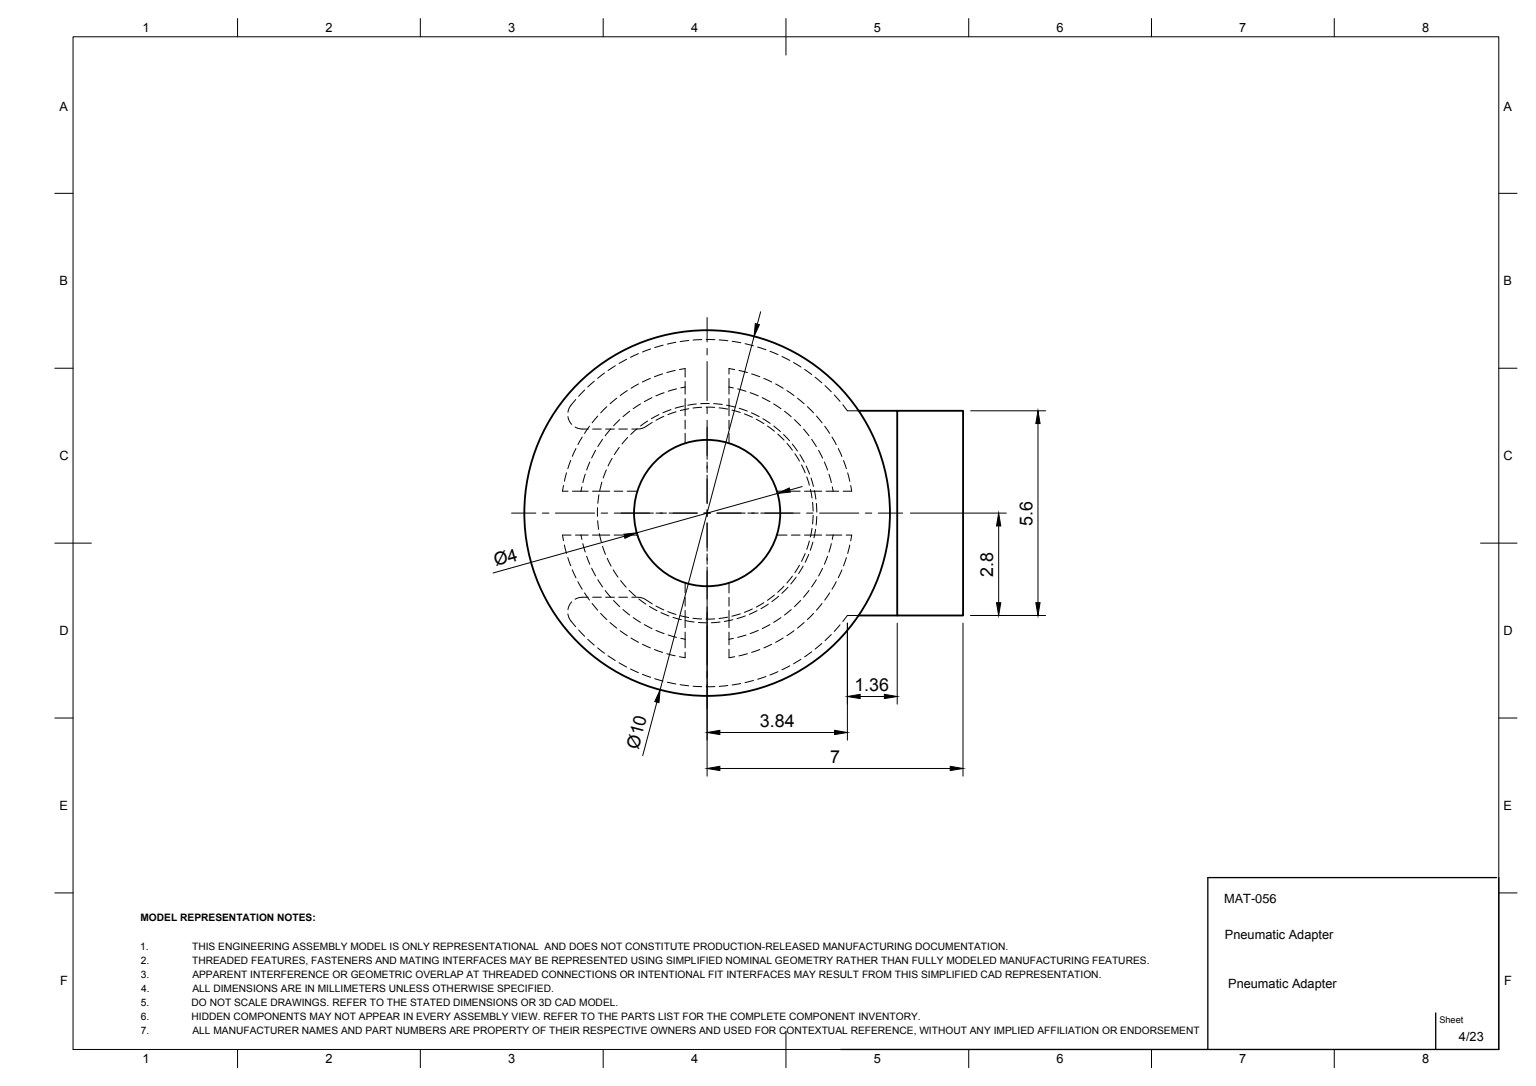
ISO-10303-21;
HEADER;
/* Generated by software containing ST-Developer
 * from STEP Tools, Inc. (www.steptools.com) 
 */

FILE_DESCRIPTION(
/* description */ (''),
/* implementation_level */ '2;1');

FILE_NAME(
/* name */ 'Pneumatic Adapter.step',
/* time_stamp */ '2026-10-28T16:47:13+01:00',
/* author */ (''),
/* organization */ (''),
/* preprocessor_version */ 'ST-DEVELOPER v20.2',
/* originating_system */ 'Autodesk Translation Framework v15.17.0.0',
/* authorisation */ '');

FILE_SCHEMA (('AUTOMOTIVE_DESIGN { 1 0 10303 214 3 1 1 }'));
ENDSEC;

DATA;
#10=MECHANICAL_DESIGN_GEOMETRIC_PRESENTATION_REPRESENTATION('',(#4567,#4568),#459242);
#4073=(
BOUNDED_CURVE()
B_SPLINE_CURVE(2,(#138438,#138439,#138440),.UNSPECIFIED.,.F.,.F.)
B_SPLINE_CURVE_WITH_KNOTS((3,3),(0.530296992815185,0.716353725522381),
 .UNSPECIFIED.)
CURVE()
GEOMETRIC_REPRESENTATION_ITEM()
RATIONAL_B_SPLINE_CURVE((1.02304101018598,1.02047479091633,1.01327152413875))
REPRESENTATION_ITEM('')
);
#4074=(
BOUNDED_CURVE()
B_SPLINE_CURVE(2,(#138443,#138444,#138445),.UNSPECIFIED.,.F.,.F.)
B_SPLINE_CURVE_WITH_KNOTS((3,3),(0.13830647491131,0.324363207617007),
 .UNSPECIFIED.)
CURVE()
GEOMETRIC_REPRESENTATION_ITEM()
RATIONAL_B_SPLINE_CURVE((1.01327152413597,1.02047479091208,1.02304101018125))
REPRESENTATION_ITEM('')
);
#4075=(
BOUNDED_CURVE()
B_SPLINE_CURVE(2,(#138448,#138449,#138450),.UNSPECIFIED.,.F.,.F.)
B_SPLINE_CURVE_WITH_KNOTS((3,3),(0.138306474911315,0.324363207616966),
 .UNSPECIFIED.)
CURVE()
GEOMETRIC_REPRESENTATION_ITEM()
RATIONAL_B_SPLINE_CURVE((1.01327152413589,1.02047479091195,1.02304101018111))
REPRESENTATION_ITEM('')
);
#4076=(
BOUNDED_CURVE()
B_SPLINE_CURVE(2,(#138452,#138453,#138454),.UNSPECIFIED.,.F.,.F.)
B_SPLINE_CURVE_WITH_KNOTS((3,3),(0.530296992818036,0.716353725523729),
 .UNSPECIFIED.)
CURVE()
GEOMETRIC_REPRESENTATION_ITEM()
RATIONAL_B_SPLINE_CURVE((1.02304101018115,1.02047479091198,1.01327152413591))
REPRESENTATION_ITEM('')
);
#4077=(
BOUNDED_CURVE()
B_SPLINE_CURVE(2,(#138458,#138459,#138460),.UNSPECIFIED.,.F.,.F.)
B_SPLINE_CURVE_WITH_KNOTS((3,3),(0.138306474911272,0.324363207616997),
 .UNSPECIFIED.)
CURVE()
GEOMETRIC_REPRESENTATION_ITEM()
RATIONAL_B_SPLINE_CURVE((1.01327152413612,1.02047479091231,1.02304101018152))
REPRESENTATION_ITEM('')
);
#4078=(
BOUNDED_CURVE()
B_SPLINE_CURVE(2,(#138462,#138463,#138464),.UNSPECIFIED.,.F.,.F.)
B_SPLINE_CURVE_WITH_KNOTS((3,3),(0.530296992818049,0.716353725523754),
 .UNSPECIFIED.)
CURVE()
GEOMETRIC_REPRESENTATION_ITEM()
RATIONAL_B_SPLINE_CURVE((1.0230410101813,1.02047479091212,1.013271524136))
REPRESENTATION_ITEM('')
);
#4079=(
BOUNDED_CURVE()
B_SPLINE_CURVE(2,(#138468,#138469,#138470),.UNSPECIFIED.,.F.,.F.)
B_SPLINE_CURVE_WITH_KNOTS((3,3),(1.87444128059995,1.89461071071013),
 .UNSPECIFIED.)
CURVE()
GEOMETRIC_REPRESENTATION_ITEM()
RATIONAL_B_SPLINE_CURVE((1.50304878048778,1.4222597775933,1.33967391292897))
REPRESENTATION_ITEM('')
);
#4080=(
BOUNDED_CURVE()
B_SPLINE_CURVE(2,(#138473,#138474,#138475),.UNSPECIFIED.,.F.,.F.)
B_SPLINE_CURVE_WITH_KNOTS((3,3),(0.0405896019330352,0.0607590320292299),
 .UNSPECIFIED.)
CURVE()
GEOMETRIC_REPRESENTATION_ITEM()
RATIONAL_B_SPLINE_CURVE((1.3396739130435,1.42225977764934,1.50304878048783))
REPRESENTATION_ITEM('')
);
#4081=(
BOUNDED_CURVE()
B_SPLINE_CURVE(2,(#138478,#138479,#138480),.UNSPECIFIED.,.F.,.F.)
B_SPLINE_CURVE_WITH_KNOTS((3,3),(0.0405896019330352,0.0607590320292299),
 .UNSPECIFIED.)
CURVE()
GEOMETRIC_REPRESENTATION_ITEM()
RATIONAL_B_SPLINE_CURVE((1.3396739130435,1.42225977764934,1.50304878048783))
REPRESENTATION_ITEM('')
);
#4082=(
BOUNDED_CURVE()
B_SPLINE_CURVE(2,(#138482,#138483,#138484),.UNSPECIFIED.,.F.,.F.)
B_SPLINE_CURVE_WITH_KNOTS((3,3),(1.87444128059996,1.89461071071012),
 .UNSPECIFIED.)
CURVE()
GEOMETRIC_REPRESENTATION_ITEM()
RATIONAL_B_SPLINE_CURVE((1.50304878048772,1.42225977759326,1.33967391292897))
REPRESENTATION_ITEM('')
);
#4083=(
BOUNDED_CURVE()
B_SPLINE_CURVE(2,(#138488,#138489,#138490),.UNSPECIFIED.,.F.,.F.)
B_SPLINE_CURVE_WITH_KNOTS((3,3),(0.0405896019330354,0.0607590320292301),
 .UNSPECIFIED.)
CURVE()
GEOMETRIC_REPRESENTATION_ITEM()
RATIONAL_B_SPLINE_CURVE((1.3396739130435,1.42225977764934,1.50304878048783))
REPRESENTATION_ITEM('')
);
#4084=(
BOUNDED_CURVE()
B_SPLINE_CURVE(2,(#138492,#138493,#138494),.UNSPECIFIED.,.F.,.F.)
B_SPLINE_CURVE_WITH_KNOTS((3,3),(1.87444128059996,1.89461071071014),
 .UNSPECIFIED.)
CURVE()
GEOMETRIC_REPRESENTATION_ITEM()
RATIONAL_B_SPLINE_CURVE((1.50304878048772,1.42225977759322,1.33967391292888))
REPRESENTATION_ITEM('')
);
#4085=(
BOUNDED_CURVE()
B_SPLINE_CURVE(2,(#138551,#138552,#138553),.UNSPECIFIED.,.F.,.F.)
B_SPLINE_CURVE_WITH_KNOTS((3,3),(0.530296992815185,0.716353725522381),
 .UNSPECIFIED.)
CURVE()
GEOMETRIC_REPRESENTATION_ITEM()
RATIONAL_B_SPLINE_CURVE((1.02304101018598,1.02047479091633,1.01327152413875))
REPRESENTATION_ITEM('')
);
#4086=(
BOUNDED_CURVE()
B_SPLINE_CURVE(2,(#138556,#138557,#138558),.UNSPECIFIED.,.F.,.F.)
B_SPLINE_CURVE_WITH_KNOTS((3,3),(0.13830647491131,0.324363207617007),
 .UNSPECIFIED.)
CURVE()
GEOMETRIC_REPRESENTATION_ITEM()
RATIONAL_B_SPLINE_CURVE((1.01327152413597,1.02047479091208,1.02304101018125))
REPRESENTATION_ITEM('')
);
#4087=(
BOUNDED_CURVE()
B_SPLINE_CURVE(2,(#138561,#138562,#138563),.UNSPECIFIED.,.F.,.F.)
B_SPLINE_CURVE_WITH_KNOTS((3,3),(1.87444128059995,1.89461071071013),
 .UNSPECIFIED.)
CURVE()
GEOMETRIC_REPRESENTATION_ITEM()
RATIONAL_B_SPLINE_CURVE((1.50304878048776,1.42225977759327,1.33967391292894))
REPRESENTATION_ITEM('')
);
#4088=(
BOUNDED_CURVE()
B_SPLINE_CURVE(2,(#138566,#138567,#138568),.UNSPECIFIED.,.F.,.F.)
B_SPLINE_CURVE_WITH_KNOTS((3,3),(0.0405896019330352,0.0607590320292299),
 .UNSPECIFIED.)
CURVE()
GEOMETRIC_REPRESENTATION_ITEM()
RATIONAL_B_SPLINE_CURVE((1.3396739130435,1.42225977764934,1.50304878048783))
REPRESENTATION_ITEM('')
);
#4406=SHAPE_REPRESENTATION_RELATIONSHIP('SRR','None',#459331,#4427);
#4427=ADVANCED_BREP_SHAPE_REPRESENTATION('',(#4448,#4449),#459220);
#4448=MANIFOLD_SOLID_BREP('Fitting body',#94624);
#4449=MANIFOLD_SOLID_BREP('Fixer',#94625);
#4567=STYLED_ITEM('',(#459519),#4448);
#4568=STYLED_ITEM('',(#459519),#4449);
#4664=CONICAL_SURFACE('',#95253,3.5,0.321750554396642);
#4665=CONICAL_SURFACE('',#95255,3.5,0.321750554396642);
#4666=CONICAL_SURFACE('',#95257,3.5,0.321750554396642);
#4667=CONICAL_SURFACE('',#95259,4.,0.558599315343569);
#4668=CONICAL_SURFACE('',#95261,4.,0.558599315343569);
#4669=CONICAL_SURFACE('',#95263,4.,0.558599315343569);
#4670=CONICAL_SURFACE('',#95281,3.5,0.321750554396642);
#4671=CONICAL_SURFACE('',#95283,4.,0.558599315343569);
#5124=FACE_BOUND('',#12374,.T.);
#5125=FACE_BOUND('',#12377,.T.);
#5321=PLANE('',#95244);
#5322=PLANE('',#95247);
#5323=PLANE('',#95250);
#5324=PLANE('',#95265);
#5325=PLANE('',#95267);
#5326=PLANE('',#95269);
#5327=PLANE('',#95279);
#5328=PLANE('',#95285);
#5329=PLANE('',#95294);
#5330=PLANE('',#95298);
#5331=PLANE('',#95299);
#5332=PLANE('',#95300);
#5333=PLANE('',#95301);
#5334=PLANE('',#95302);
#5335=PLANE('',#95303);
#5336=PLANE('',#95304);
#5337=PLANE('',#95305);
#5338=PLANE('',#95306);
#5339=PLANE('',#95307);
#5340=PLANE('',#95308);
#5341=PLANE('',#95309);
#5342=PLANE('',#95310);
#5343=PLANE('',#95314);
#5344=PLANE('',#95315);
#5345=PLANE('',#95334);
#5346=PLANE('',#95335);
#5347=PLANE('',#95336);
#5348=PLANE('',#95337);
#5349=PLANE('',#95338);
#5350=PLANE('',#95339);
#5351=PLANE('',#95340);
#6536=FACE_OUTER_BOUND('',#12355,.T.);
#6537=FACE_OUTER_BOUND('',#12356,.T.);
#6538=FACE_OUTER_BOUND('',#12357,.T.);
#6539=FACE_OUTER_BOUND('',#12358,.T.);
#6540=FACE_OUTER_BOUND('',#12359,.T.);
#6541=FACE_OUTER_BOUND('',#12360,.T.);
#6542=FACE_OUTER_BOUND('',#12361,.T.);
#6543=FACE_OUTER_BOUND('',#12362,.T.);
#6544=FACE_OUTER_BOUND('',#12363,.T.);
#6545=FACE_OUTER_BOUND('',#12364,.T.);
#6546=FACE_OUTER_BOUND('',#12365,.T.);
#6547=FACE_OUTER_BOUND('',#12366,.T.);
#6548=FACE_OUTER_BOUND('',#12367,.T.);
#6549=FACE_OUTER_BOUND('',#12368,.T.);
#6550=FACE_OUTER_BOUND('',#12369,.T.);
#6551=FACE_OUTER_BOUND('',#12370,.T.);
#6552=FACE_OUTER_BOUND('',#12371,.T.);
#6553=FACE_OUTER_BOUND('',#12372,.T.);
#6554=FACE_OUTER_BOUND('',#12373,.T.);
#6555=FACE_OUTER_BOUND('',#12375,.T.);
#6556=FACE_OUTER_BOUND('',#12376,.T.);
#6557=FACE_OUTER_BOUND('',#12378,.T.);
#6558=FACE_OUTER_BOUND('',#12379,.T.);
#6559=FACE_OUTER_BOUND('',#12380,.T.);
#6560=FACE_OUTER_BOUND('',#12381,.T.);
#6561=FACE_OUTER_BOUND('',#12382,.T.);
#6562=FACE_OUTER_BOUND('',#12383,.T.);
#6563=FACE_OUTER_BOUND('',#12384,.T.);
#6564=FACE_OUTER_BOUND('',#12385,.T.);
#6565=FACE_OUTER_BOUND('',#12386,.T.);
#6566=FACE_OUTER_BOUND('',#12387,.T.);
#6567=FACE_OUTER_BOUND('',#12388,.T.);
#6568=FACE_OUTER_BOUND('',#12389,.T.);
#6569=FACE_OUTER_BOUND('',#12390,.T.);
#6570=FACE_OUTER_BOUND('',#12391,.T.);
#6571=FACE_OUTER_BOUND('',#12392,.T.);
#6572=FACE_OUTER_BOUND('',#12393,.T.);
#6573=FACE_OUTER_BOUND('',#12394,.T.);
#6574=FACE_OUTER_BOUND('',#12395,.T.);
#6575=FACE_OUTER_BOUND('',#12396,.T.);
#6576=FACE_OUTER_BOUND('',#12397,.T.);
#6577=FACE_OUTER_BOUND('',#12398,.T.);
#6578=FACE_OUTER_BOUND('',#12399,.T.);
#6579=FACE_OUTER_BOUND('',#12400,.T.);
#6580=FACE_OUTER_BOUND('',#12401,.T.);
#6581=FACE_OUTER_BOUND('',#12402,.T.);
#6582=FACE_OUTER_BOUND('',#12403,.T.);
#6583=FACE_OUTER_BOUND('',#12404,.T.);
#6584=FACE_OUTER_BOUND('',#12405,.T.);
#12355=EDGE_LOOP('',(#59046,#59047,#59048,#59049));
#12356=EDGE_LOOP('',(#59050,#59051,#59052,#59053));
#12357=EDGE_LOOP('',(#59054,#59055,#59056,#59057));
#12358=EDGE_LOOP('',(#59058,#59059,#59060,#59061));
#12359=EDGE_LOOP('',(#59062,#59063,#59064,#59065));
#12360=EDGE_LOOP('',(#59066,#59067,#59068,#59069));
#12361=EDGE_LOOP('',(#59070,#59071,#59072,#59073));
#12362=EDGE_LOOP('',(#59074,#59075,#59076,#59077));
#12363=EDGE_LOOP('',(#59078,#59079,#59080,#59081));
#12364=EDGE_LOOP('',(#59082,#59083,#59084,#59085));
#12365=EDGE_LOOP('',(#59086,#59087,#59088,#59089));
#12366=EDGE_LOOP('',(#59090,#59091,#59092,#59093));
#12367=EDGE_LOOP('',(#59094,#59095,#59096,#59097,#59098,#59099,#59100,#59101,
#59102,#59103,#59104,#59105,#59106,#59107,#59108,#59109,#59110,#59111,#59112,
#59113));
#12368=EDGE_LOOP('',(#59114,#59115,#59116,#59117));
#12369=EDGE_LOOP('',(#59118,#59119,#59120,#59121));
#12370=EDGE_LOOP('',(#59122,#59123,#59124,#59125));
#12371=EDGE_LOOP('',(#59126,#59127,#59128,#59129));
#12372=EDGE_LOOP('',(#59130,#59131,#59132,#59133,#59134,#59135,#59136,#59137,
#59138,#59139,#59140,#59141,#59142,#59143,#59144,#59145,#59146,#59147,#59148,
#59149));
#12373=EDGE_LOOP('',(#59150));
#12374=EDGE_LOOP('',(#59151));
#12375=EDGE_LOOP('',(#59152,#59153,#59154,#59155));
#12376=EDGE_LOOP('',(#59156));
#12377=EDGE_LOOP('',(#59157));
#12378=EDGE_LOOP('',(#59158,#59159,#59160,#59161,#59162,#59163,#59164));
#12379=EDGE_LOOP('',(#59165,#59166,#59167,#59168,#59169,#59170,#59171));
#12380=EDGE_LOOP('',(#59172,#59173,#59174,#59175,#59176,#59177));
#12381=EDGE_LOOP('',(#59178,#59179,#59180,#59181,#59182,#59183,#59184));
#12382=EDGE_LOOP('',(#59185,#59186,#59187,#59188,#59189,#59190,#59191));
#12383=EDGE_LOOP('',(#59192,#59193,#59194,#59195));
#12384=EDGE_LOOP('',(#59196,#59197,#59198,#59199,#59200,#59201,#59202));
#12385=EDGE_LOOP('',(#59203,#59204,#59205,#59206,#59207,#59208,#59209));
#12386=EDGE_LOOP('',(#59210,#59211,#59212,#59213));
#12387=EDGE_LOOP('',(#59214,#59215,#59216,#59217,#59218,#59219,#59220));
#12388=EDGE_LOOP('',(#59221,#59222,#59223,#59224,#59225,#59226,#59227));
#12389=EDGE_LOOP('',(#59228,#59229,#59230,#59231));
#12390=EDGE_LOOP('',(#59232,#59233,#59234,#59235));
#12391=EDGE_LOOP('',(#59236,#59237,#59238,#59239));
#12392=EDGE_LOOP('',(#59240,#59241,#59242,#59243,#59244,#59245,#59246,#59247,
#59248,#59249,#59250,#59251));
#12393=EDGE_LOOP('',(#59252,#59253,#59254,#59255));
#12394=EDGE_LOOP('',(#59256,#59257,#59258,#59259));
#12395=EDGE_LOOP('',(#59260,#59261,#59262,#59263));
#12396=EDGE_LOOP('',(#59264,#59265,#59266,#59267));
#12397=EDGE_LOOP('',(#59268,#59269,#59270,#59271));
#12398=EDGE_LOOP('',(#59272,#59273,#59274,#59275));
#12399=EDGE_LOOP('',(#59276,#59277,#59278,#59279));
#12400=EDGE_LOOP('',(#59280,#59281,#59282,#59283));
#12401=EDGE_LOOP('',(#59284,#59285,#59286,#59287));
#12402=EDGE_LOOP('',(#59288,#59289,#59290,#59291,#59292,#59293));
#12403=EDGE_LOOP('',(#59294,#59295,#59296,#59297));
#12404=EDGE_LOOP('',(#59298,#59299,#59300,#59301,#59302,#59303));
#12405=EDGE_LOOP('',(#59304,#59305,#59306,#59307,#59308,#59309,#59310,#59311,
#59312,#59313,#59314,#59315));
#18307=CIRCLE('',#95245,3.5);
#18308=CIRCLE('',#95246,2.);
#18309=CIRCLE('',#95248,2.);
#18310=CIRCLE('',#95249,3.5);
#18311=CIRCLE('',#95251,2.);
#18312=CIRCLE('',#95252,3.5);
#18313=CIRCLE('',#95254,4.);
#18314=CIRCLE('',#95256,4.);
#18315=CIRCLE('',#95258,4.);
#18316=CIRCLE('',#95260,3.49999999999999);
#18317=CIRCLE('',#95262,3.49999999999999);
#18318=CIRCLE('',#95264,3.49999999999999);
#18319=CIRCLE('',#95266,3.);
#18320=CIRCLE('',#95268,3.);
#18321=CIRCLE('',#95270,3.);
#18322=CIRCLE('',#95272,2.);
#18323=CIRCLE('',#95273,2.);
#18324=CIRCLE('',#95274,2.);
#18325=CIRCLE('',#95275,2.);
#18326=CIRCLE('',#95276,2.);
#18327=CIRCLE('',#95277,2.);
#18328=CIRCLE('',#95278,2.);
#18329=CIRCLE('',#95280,3.5);
#18330=CIRCLE('',#95282,4.);
#18331=CIRCLE('',#95284,3.49999999999999);
#18332=CIRCLE('',#95286,3.);
#18333=CIRCLE('',#95288,3.);
#18334=CIRCLE('',#95289,3.);
#18335=CIRCLE('',#95290,3.);
#18336=CIRCLE('',#95291,3.);
#18337=CIRCLE('',#95292,3.);
#18338=CIRCLE('',#95293,3.);
#18339=CIRCLE('',#95295,5.);
#18340=CIRCLE('',#95297,5.);
#18341=CIRCLE('',#95312,0.4);
#18342=CIRCLE('',#95313,0.4);
#18343=CIRCLE('',#95316,2.9);
#18344=CIRCLE('',#95317,0.4);
#18345=CIRCLE('',#95318,0.4);
#18346=CIRCLE('',#95319,4.75);
#18347=CIRCLE('',#95320,4.75);
#18348=CIRCLE('',#95321,0.4);
#18349=CIRCLE('',#95323,0.4);
#18350=CIRCLE('',#95325,4.75);
#18351=CIRCLE('',#95327,0.4);
#18352=CIRCLE('',#95329,2.9);
#18353=CIRCLE('',#95331,0.4);
#18354=CIRCLE('',#95333,4.75);
#27269=LINE('',#138412,#31071);
#27270=LINE('',#138416,#31072);
#27271=LINE('',#138421,#31073);
#27272=LINE('',#138425,#31074);
#27273=LINE('',#138430,#31075);
#27274=LINE('',#138434,#31076);
#27275=LINE('',#138498,#31077);
#27276=LINE('',#138501,#31078);
#27277=LINE('',#138504,#31079);
#27278=LINE('',#138506,#31080);
#27279=LINE('',#138510,#31081);
#27280=LINE('',#138512,#31082);
#27281=LINE('',#138518,#31083);
#27282=LINE('',#138521,#31084);
#27283=LINE('',#138523,#31085);
#27284=LINE('',#138526,#31086);
#27285=LINE('',#138528,#31087);
#27286=LINE('',#138531,#31088);
#27287=LINE('',#138533,#31089);
#27288=LINE('',#138537,#31090);
#27289=LINE('',#138541,#31091);
#27290=LINE('',#138545,#31092);
#27291=LINE('',#138548,#31093);
#27292=LINE('',#138571,#31094);
#27293=LINE('',#138574,#31095);
#27294=LINE('',#138580,#31096);
#27295=LINE('',#138584,#31097);
#27296=LINE('',#138586,#31098);
#27297=LINE('',#138589,#31099);
#27298=LINE('',#138591,#31100);
#27299=LINE('',#138594,#31101);
#27300=LINE('',#138596,#31102);
#27301=LINE('',#138599,#31103);
#27302=LINE('',#138600,#31104);
#27303=LINE('',#138606,#31105);
#27304=LINE('',#138610,#31106);
#27305=LINE('',#138612,#31107);
#27306=LINE('',#138615,#31108);
#27307=LINE('',#138617,#31109);
#27308=LINE('',#138620,#31110);
#27309=LINE('',#138622,#31111);
#27310=LINE('',#138625,#31112);
#27311=LINE('',#138627,#31113);
#27312=LINE('',#138634,#31114);
#27313=LINE('',#138637,#31115);
#27314=LINE('',#138640,#31116);
#27315=LINE('',#138642,#31117);
#27316=LINE('',#138643,#31118);
#27317=LINE('',#138650,#31119);
#27318=LINE('',#138656,#31120);
#27319=LINE('',#138658,#31121);
#27320=LINE('',#138660,#31122);
#27321=LINE('',#138667,#31123);
#27322=LINE('',#138670,#31124);
#27323=LINE('',#138676,#31125);
#27324=LINE('',#138677,#31126);
#27325=LINE('',#138684,#31127);
#27326=LINE('',#138685,#31128);
#27327=LINE('',#138689,#31129);
#27328=LINE('',#138692,#31130);
#27329=LINE('',#138694,#31131);
#27330=LINE('',#138695,#31132);
#27331=LINE('',#138698,#31133);
#27332=LINE('',#138700,#31134);
#27333=LINE('',#138701,#31135);
#27334=LINE('',#138704,#31136);
#27335=LINE('',#138706,#31137);
#27336=LINE('',#138707,#31138);
#27337=LINE('',#138709,#31139);
#27338=LINE('',#138711,#31140);
#27339=LINE('',#138713,#31141);
#31071=VECTOR('',#106479,1000.);
#31072=VECTOR('',#106482,1000.);
#31073=VECTOR('',#106487,1000.);
#31074=VECTOR('',#106490,1000.);
#31075=VECTOR('',#106495,1000.);
#31076=VECTOR('',#106498,1000.);
#31077=VECTOR('',#106527,1000.);
#31078=VECTOR('',#106530,1000.);
#31079=VECTOR('',#106533,1000.);
#31080=VECTOR('',#106534,1000.);
#31081=VECTOR('',#106539,1000.);
#31082=VECTOR('',#106540,1000.);
#31083=VECTOR('',#106547,2.);
#31084=VECTOR('',#106550,1000.);
#31085=VECTOR('',#106551,1000.);
#31086=VECTOR('',#106554,1000.);
#31087=VECTOR('',#106555,1000.);
#31088=VECTOR('',#106558,1000.);
#31089=VECTOR('',#106559,1000.);
#31090=VECTOR('',#106562,1000.);
#31091=VECTOR('',#106565,1000.);
#31092=VECTOR('',#106570,1000.);
#31093=VECTOR('',#106573,1000.);
#31094=VECTOR('',#106584,1000.);
#31095=VECTOR('',#106587,1000.);
#31096=VECTOR('',#106592,3.);
#31097=VECTOR('',#106597,1000.);
#31098=VECTOR('',#106598,1000.);
#31099=VECTOR('',#106601,1000.);
#31100=VECTOR('',#106602,1000.);
#31101=VECTOR('',#106605,1000.);
#31102=VECTOR('',#106606,1000.);
#31103=VECTOR('',#106609,1000.);
#31104=VECTOR('',#106610,1000.);
#31105=VECTOR('',#106617,5.);
#31106=VECTOR('',#106624,1000.);
#31107=VECTOR('',#106627,1000.);
#31108=VECTOR('',#106632,1000.);
#31109=VECTOR('',#106635,1000.);
#31110=VECTOR('',#106640,1000.);
#31111=VECTOR('',#106643,1000.);
#31112=VECTOR('',#106648,1000.);
#31113=VECTOR('',#106651,1000.);
#31114=VECTOR('',#106658,10.);
#31115=VECTOR('',#106661,10.);
#31116=VECTOR('',#106664,10.);
#31117=VECTOR('',#106665,10.);
#31118=VECTOR('',#106666,10.);
#31119=VECTOR('',#106673,10.);
#31120=VECTOR('',#106678,10.);
#31121=VECTOR('',#106679,10.);
#31122=VECTOR('',#106680,10.);
#31123=VECTOR('',#106689,10.);
#31124=VECTOR('',#106692,10.);
#31125=VECTOR('',#106699,10.);
#31126=VECTOR('',#106700,10.);
#31127=VECTOR('',#106709,10.);
#31128=VECTOR('',#106710,10.);
#31129=VECTOR('',#106715,10.);
#31130=VECTOR('',#106718,10.);
#31131=VECTOR('',#106719,10.);
#31132=VECTOR('',#106720,10.);
#31133=VECTOR('',#106723,10.);
#31134=VECTOR('',#106724,10.);
#31135=VECTOR('',#106725,10.);
#31136=VECTOR('',#106728,10.);
#31137=VECTOR('',#106729,10.);
#31138=VECTOR('',#106730,10.);
#31139=VECTOR('',#106733,10.);
#31140=VECTOR('',#106736,10.);
#31141=VECTOR('',#106739,10.);
#34984=VERTEX_POINT('',#138410);
#34985=VERTEX_POINT('',#138411);
#34986=VERTEX_POINT('',#138413);
#34987=VERTEX_POINT('',#138415);
#34988=VERTEX_POINT('',#138419);
#34989=VERTEX_POINT('',#138420);
#34990=VERTEX_POINT('',#138422);
#34991=VERTEX_POINT('',#138424);
#34992=VERTEX_POINT('',#138428);
#34993=VERTEX_POINT('',#138429);
#34994=VERTEX_POINT('',#138431);
#34995=VERTEX_POINT('',#138433);
#34996=VERTEX_POINT('',#138437);
#34997=VERTEX_POINT('',#138441);
#34998=VERTEX_POINT('',#138447);
#34999=VERTEX_POINT('',#138451);
#35000=VERTEX_POINT('',#138457);
#35001=VERTEX_POINT('',#138461);
#35002=VERTEX_POINT('',#138467);
#35003=VERTEX_POINT('',#138471);
#35004=VERTEX_POINT('',#138477);
#35005=VERTEX_POINT('',#138481);
#35006=VERTEX_POINT('',#138487);
#35007=VERTEX_POINT('',#138491);
#35008=VERTEX_POINT('',#138497);
#35009=VERTEX_POINT('',#138499);
#35010=VERTEX_POINT('',#138503);
#35011=VERTEX_POINT('',#138505);
#35012=VERTEX_POINT('',#138509);
#35013=VERTEX_POINT('',#138511);
#35014=VERTEX_POINT('',#138515);
#35015=VERTEX_POINT('',#138517);
#35016=VERTEX_POINT('',#138519);
#35017=VERTEX_POINT('',#138522);
#35018=VERTEX_POINT('',#138524);
#35019=VERTEX_POINT('',#138527);
#35020=VERTEX_POINT('',#138529);
#35021=VERTEX_POINT('',#138532);
#35022=VERTEX_POINT('',#138534);
#35023=VERTEX_POINT('',#138536);
#35024=VERTEX_POINT('',#138538);
#35025=VERTEX_POINT('',#138540);
#35026=VERTEX_POINT('',#138544);
#35027=VERTEX_POINT('',#138546);
#35028=VERTEX_POINT('',#138550);
#35029=VERTEX_POINT('',#138554);
#35030=VERTEX_POINT('',#138560);
#35031=VERTEX_POINT('',#138564);
#35032=VERTEX_POINT('',#138570);
#35033=VERTEX_POINT('',#138572);
#35034=VERTEX_POINT('',#138576);
#35035=VERTEX_POINT('',#138577);
#35036=VERTEX_POINT('',#138579);
#35037=VERTEX_POINT('',#138582);
#35038=VERTEX_POINT('',#138585);
#35039=VERTEX_POINT('',#138587);
#35040=VERTEX_POINT('',#138590);
#35041=VERTEX_POINT('',#138592);
#35042=VERTEX_POINT('',#138595);
#35043=VERTEX_POINT('',#138597);
#35044=VERTEX_POINT('',#138602);
#35045=VERTEX_POINT('',#138605);
#35046=VERTEX_POINT('',#138630);
#35047=VERTEX_POINT('',#138631);
#35048=VERTEX_POINT('',#138633);
#35049=VERTEX_POINT('',#138635);
#35050=VERTEX_POINT('',#138639);
#35051=VERTEX_POINT('',#138641);
#35052=VERTEX_POINT('',#138645);
#35053=VERTEX_POINT('',#138647);
#35054=VERTEX_POINT('',#138649);
#35055=VERTEX_POINT('',#138651);
#35056=VERTEX_POINT('',#138653);
#35057=VERTEX_POINT('',#138655);
#35058=VERTEX_POINT('',#138657);
#35059=VERTEX_POINT('',#138659);
#35060=VERTEX_POINT('',#138661);
#35061=VERTEX_POINT('',#138665);
#35062=VERTEX_POINT('',#138669);
#35063=VERTEX_POINT('',#138673);
#35064=VERTEX_POINT('',#138674);
#35065=VERTEX_POINT('',#138681);
#35066=VERTEX_POINT('',#138682);
#35067=VERTEX_POINT('',#138687);
#35068=VERTEX_POINT('',#138691);
#35069=VERTEX_POINT('',#138693);
#35070=VERTEX_POINT('',#138697);
#35071=VERTEX_POINT('',#138699);
#35072=VERTEX_POINT('',#138703);
#35073=VERTEX_POINT('',#138705);
#44025=EDGE_CURVE('',#34984,#34985,#27269,.T.);
#44026=EDGE_CURVE('',#34984,#34986,#18307,.T.);
#44027=EDGE_CURVE('',#34987,#34986,#27270,.T.);
#44028=EDGE_CURVE('',#34985,#34987,#18308,.T.);
#44029=EDGE_CURVE('',#34988,#34989,#27271,.T.);
#44030=EDGE_CURVE('',#34990,#34988,#18309,.T.);
#44031=EDGE_CURVE('',#34991,#34990,#27272,.T.);
#44032=EDGE_CURVE('',#34991,#34989,#18310,.T.);
#44033=EDGE_CURVE('',#34992,#34993,#27273,.T.);
#44034=EDGE_CURVE('',#34994,#34992,#18311,.T.);
#44035=EDGE_CURVE('',#34995,#34994,#27274,.T.);
#44036=EDGE_CURVE('',#34995,#34993,#18312,.T.);
#44037=EDGE_CURVE('',#34996,#34984,#4073,.T.);
#44038=EDGE_CURVE('',#34996,#34997,#18313,.T.);
#44039=EDGE_CURVE('',#34986,#34997,#4074,.T.);
#44040=EDGE_CURVE('',#34989,#34998,#4075,.T.);
#44041=EDGE_CURVE('',#34999,#34991,#4076,.T.);
#44042=EDGE_CURVE('',#34999,#34998,#18314,.T.);
#44043=EDGE_CURVE('',#34993,#35000,#4077,.T.);
#44044=EDGE_CURVE('',#35001,#34995,#4078,.T.);
#44045=EDGE_CURVE('',#35001,#35000,#18315,.T.);
#44046=EDGE_CURVE('',#35002,#34996,#4079,.T.);
#44047=EDGE_CURVE('',#35002,#35003,#18316,.T.);
#44048=EDGE_CURVE('',#34997,#35003,#4080,.T.);
#44049=EDGE_CURVE('',#34998,#35004,#4081,.T.);
#44050=EDGE_CURVE('',#35005,#34999,#4082,.T.);
#44051=EDGE_CURVE('',#35005,#35004,#18317,.T.);
#44052=EDGE_CURVE('',#35000,#35006,#4083,.T.);
#44053=EDGE_CURVE('',#35007,#35001,#4084,.T.);
#44054=EDGE_CURVE('',#35007,#35006,#18318,.T.);
#44055=EDGE_CURVE('',#35008,#35002,#27275,.T.);
#44056=EDGE_CURVE('',#35008,#35009,#18319,.T.);
#44057=EDGE_CURVE('',#35003,#35009,#27276,.T.);
#44058=EDGE_CURVE('',#35004,#35010,#27277,.T.);
#44059=EDGE_CURVE('',#35011,#35005,#27278,.T.);
#44060=EDGE_CURVE('',#35011,#35010,#18320,.T.);
#44061=EDGE_CURVE('',#35006,#35012,#27279,.T.);
#44062=EDGE_CURVE('',#35013,#35007,#27280,.T.);
#44063=EDGE_CURVE('',#35013,#35012,#18321,.T.);
#44064=EDGE_CURVE('',#35014,#35014,#18322,.T.);
#44065=EDGE_CURVE('',#35014,#35015,#27281,.T.);
#44066=EDGE_CURVE('',#35015,#35016,#18323,.T.);
#44067=EDGE_CURVE('',#35016,#34994,#27282,.T.);
#44068=EDGE_CURVE('',#35017,#34992,#27283,.T.);
#44069=EDGE_CURVE('',#35017,#35018,#18324,.T.);
#44070=EDGE_CURVE('',#35018,#34990,#27284,.T.);
#44071=EDGE_CURVE('',#35019,#34988,#27285,.T.);
#44072=EDGE_CURVE('',#35019,#35020,#18325,.T.);
#44073=EDGE_CURVE('',#35020,#34985,#27286,.T.);
#44074=EDGE_CURVE('',#35021,#34987,#27287,.T.);
#44075=EDGE_CURVE('',#35021,#35022,#18326,.T.);
#44076=EDGE_CURVE('',#35022,#35023,#27288,.T.);
#44077=EDGE_CURVE('',#35023,#35024,#18327,.T.);
#44078=EDGE_CURVE('',#35025,#35024,#27289,.T.);
#44079=EDGE_CURVE('',#35025,#35015,#18328,.T.);
#44080=EDGE_CURVE('',#35026,#35023,#27290,.T.);
#44081=EDGE_CURVE('',#35026,#35027,#18329,.T.);
#44082=EDGE_CURVE('',#35024,#35027,#27291,.T.);
#44083=EDGE_CURVE('',#35028,#35026,#4085,.T.);
#44084=EDGE_CURVE('',#35028,#35029,#18330,.T.);
#44085=EDGE_CURVE('',#35027,#35029,#4086,.T.);
#44086=EDGE_CURVE('',#35030,#35028,#4087,.T.);
#44087=EDGE_CURVE('',#35030,#35031,#18331,.T.);
#44088=EDGE_CURVE('',#35029,#35031,#4088,.T.);
#44089=EDGE_CURVE('',#35032,#35030,#27292,.T.);
#44090=EDGE_CURVE('',#35032,#35033,#18332,.T.);
#44091=EDGE_CURVE('',#35031,#35033,#27293,.T.);
#44092=EDGE_CURVE('',#35034,#35035,#18333,.F.);
#44093=EDGE_CURVE('',#35035,#35036,#27294,.T.);
#44094=EDGE_CURVE('',#35036,#35036,#18334,.T.);
#44095=EDGE_CURVE('',#35035,#35037,#18335,.F.);
#44096=EDGE_CURVE('',#35033,#35037,#27295,.F.);
#44097=EDGE_CURVE('',#35038,#35032,#27296,.T.);
#44098=EDGE_CURVE('',#35038,#35039,#18336,.F.);
#44099=EDGE_CURVE('',#35009,#35039,#27297,.F.);
#44100=EDGE_CURVE('',#35040,#35008,#27298,.T.);
#44101=EDGE_CURVE('',#35040,#35041,#18337,.F.);
#44102=EDGE_CURVE('',#35010,#35041,#27299,.F.);
#44103=EDGE_CURVE('',#35042,#35011,#27300,.T.);
#44104=EDGE_CURVE('',#35042,#35043,#18338,.F.);
#44105=EDGE_CURVE('',#35012,#35043,#27301,.F.);
#44106=EDGE_CURVE('',#35034,#35013,#27302,.T.);
#44107=EDGE_CURVE('',#35044,#35044,#18339,.T.);
#44108=EDGE_CURVE('',#35044,#35045,#27303,.T.);
#44109=EDGE_CURVE('',#35045,#35045,#18340,.T.);
#44110=EDGE_CURVE('',#35037,#35025,#27304,.F.);
#44111=EDGE_CURVE('',#35016,#35034,#27305,.F.);
#44112=EDGE_CURVE('',#35039,#35021,#27306,.F.);
#44113=EDGE_CURVE('',#35022,#35038,#27307,.F.);
#44114=EDGE_CURVE('',#35018,#35042,#27308,.F.);
#44115=EDGE_CURVE('',#35043,#35017,#27309,.F.);
#44116=EDGE_CURVE('',#35020,#35040,#27310,.F.);
#44117=EDGE_CURVE('',#35041,#35019,#27311,.F.);
#44118=EDGE_CURVE('',#35046,#35047,#18341,.T.);
#44119=EDGE_CURVE('',#35047,#35048,#27312,.T.);
#44120=EDGE_CURVE('',#35048,#35049,#18342,.T.);
#44121=EDGE_CURVE('',#35049,#35046,#27313,.T.);
#44122=EDGE_CURVE('',#35049,#35050,#27314,.T.);
#44123=EDGE_CURVE('',#35051,#35050,#27315,.T.);
#44124=EDGE_CURVE('',#35046,#35051,#27316,.T.);
#44125=EDGE_CURVE('',#35048,#35052,#18343,.T.);
#44126=EDGE_CURVE('',#35053,#35052,#18344,.T.);
#44127=EDGE_CURVE('',#35053,#35054,#27317,.T.);
#44128=EDGE_CURVE('',#35055,#35054,#18345,.T.);
#44129=EDGE_CURVE('',#35056,#35055,#18346,.T.);
#44130=EDGE_CURVE('',#35057,#35056,#27318,.T.);
#44131=EDGE_CURVE('',#35057,#35058,#27319,.T.);
#44132=EDGE_CURVE('',#35058,#35059,#27320,.T.);
#44133=EDGE_CURVE('',#35060,#35059,#18347,.T.);
#44134=EDGE_CURVE('',#35050,#35060,#18348,.T.);
#44135=EDGE_CURVE('',#35061,#35051,#18349,.T.);
#44136=EDGE_CURVE('',#35060,#35061,#27321,.T.);
#44137=EDGE_CURVE('',#35059,#35062,#27322,.T.);
#44138=EDGE_CURVE('',#35061,#35062,#18350,.T.);
#44139=EDGE_CURVE('',#35063,#35064,#18351,.T.);
#44140=EDGE_CURVE('',#35064,#35053,#27323,.T.);
#44141=EDGE_CURVE('',#35052,#35063,#27324,.T.);
#44142=EDGE_CURVE('',#35063,#35047,#18352,.T.);
#44143=EDGE_CURVE('',#35065,#35066,#18353,.T.);
#44144=EDGE_CURVE('',#35066,#35055,#27325,.T.);
#44145=EDGE_CURVE('',#35054,#35065,#27326,.T.);
#44146=EDGE_CURVE('',#35067,#35066,#18354,.T.);
#44147=EDGE_CURVE('',#35056,#35067,#27327,.T.);
#44148=EDGE_CURVE('',#35057,#35068,#27328,.T.);
#44149=EDGE_CURVE('',#35069,#35068,#27329,.T.);
#44150=EDGE_CURVE('',#35058,#35069,#27330,.T.);
#44151=EDGE_CURVE('',#35068,#35070,#27331,.T.);
#44152=EDGE_CURVE('',#35070,#35071,#27332,.T.);
#44153=EDGE_CURVE('',#35071,#35069,#27333,.T.);
#44154=EDGE_CURVE('',#35072,#35070,#27334,.T.);
#44155=EDGE_CURVE('',#35073,#35072,#27335,.T.);
#44156=EDGE_CURVE('',#35071,#35073,#27336,.T.);
#44157=EDGE_CURVE('',#35062,#35073,#27337,.T.);
#44158=EDGE_CURVE('',#35065,#35064,#27338,.T.);
#44159=EDGE_CURVE('',#35072,#35067,#27339,.T.);
#59046=ORIENTED_EDGE('',*,*,#44025,.F.);
#59047=ORIENTED_EDGE('',*,*,#44026,.T.);
#59048=ORIENTED_EDGE('',*,*,#44027,.F.);
#59049=ORIENTED_EDGE('',*,*,#44028,.F.);
#59050=ORIENTED_EDGE('',*,*,#44029,.F.);
#59051=ORIENTED_EDGE('',*,*,#44030,.F.);
#59052=ORIENTED_EDGE('',*,*,#44031,.F.);
#59053=ORIENTED_EDGE('',*,*,#44032,.T.);
#59054=ORIENTED_EDGE('',*,*,#44033,.F.);
#59055=ORIENTED_EDGE('',*,*,#44034,.F.);
#59056=ORIENTED_EDGE('',*,*,#44035,.F.);
#59057=ORIENTED_EDGE('',*,*,#44036,.T.);
#59058=ORIENTED_EDGE('',*,*,#44037,.F.);
#59059=ORIENTED_EDGE('',*,*,#44038,.T.);
#59060=ORIENTED_EDGE('',*,*,#44039,.F.);
#59061=ORIENTED_EDGE('',*,*,#44026,.F.);
#59062=ORIENTED_EDGE('',*,*,#44040,.F.);
#59063=ORIENTED_EDGE('',*,*,#44032,.F.);
#59064=ORIENTED_EDGE('',*,*,#44041,.F.);
#59065=ORIENTED_EDGE('',*,*,#44042,.T.);
#59066=ORIENTED_EDGE('',*,*,#44043,.F.);
#59067=ORIENTED_EDGE('',*,*,#44036,.F.);
#59068=ORIENTED_EDGE('',*,*,#44044,.F.);
#59069=ORIENTED_EDGE('',*,*,#44045,.T.);
#59070=ORIENTED_EDGE('',*,*,#44046,.F.);
#59071=ORIENTED_EDGE('',*,*,#44047,.T.);
#59072=ORIENTED_EDGE('',*,*,#44048,.F.);
#59073=ORIENTED_EDGE('',*,*,#44038,.F.);
#59074=ORIENTED_EDGE('',*,*,#44049,.F.);
#59075=ORIENTED_EDGE('',*,*,#44042,.F.);
#59076=ORIENTED_EDGE('',*,*,#44050,.F.);
#59077=ORIENTED_EDGE('',*,*,#44051,.T.);
#59078=ORIENTED_EDGE('',*,*,#44052,.F.);
#59079=ORIENTED_EDGE('',*,*,#44045,.F.);
#59080=ORIENTED_EDGE('',*,*,#44053,.F.);
#59081=ORIENTED_EDGE('',*,*,#44054,.T.);
#59082=ORIENTED_EDGE('',*,*,#44055,.F.);
#59083=ORIENTED_EDGE('',*,*,#44056,.T.);
#59084=ORIENTED_EDGE('',*,*,#44057,.F.);
#59085=ORIENTED_EDGE('',*,*,#44047,.F.);
#59086=ORIENTED_EDGE('',*,*,#44058,.F.);
#59087=ORIENTED_EDGE('',*,*,#44051,.F.);
#59088=ORIENTED_EDGE('',*,*,#44059,.F.);
#59089=ORIENTED_EDGE('',*,*,#44060,.T.);
#59090=ORIENTED_EDGE('',*,*,#44061,.F.);
#59091=ORIENTED_EDGE('',*,*,#44054,.F.);
#59092=ORIENTED_EDGE('',*,*,#44062,.F.);
#59093=ORIENTED_EDGE('',*,*,#44063,.T.);
#59094=ORIENTED_EDGE('',*,*,#44064,.F.);
#59095=ORIENTED_EDGE('',*,*,#44065,.T.);
#59096=ORIENTED_EDGE('',*,*,#44066,.T.);
#59097=ORIENTED_EDGE('',*,*,#44067,.T.);
#59098=ORIENTED_EDGE('',*,*,#44034,.T.);
#59099=ORIENTED_EDGE('',*,*,#44068,.F.);
#59100=ORIENTED_EDGE('',*,*,#44069,.T.);
#59101=ORIENTED_EDGE('',*,*,#44070,.T.);
#59102=ORIENTED_EDGE('',*,*,#44030,.T.);
#59103=ORIENTED_EDGE('',*,*,#44071,.F.);
#59104=ORIENTED_EDGE('',*,*,#44072,.T.);
#59105=ORIENTED_EDGE('',*,*,#44073,.T.);
#59106=ORIENTED_EDGE('',*,*,#44028,.T.);
#59107=ORIENTED_EDGE('',*,*,#44074,.F.);
#59108=ORIENTED_EDGE('',*,*,#44075,.T.);
#59109=ORIENTED_EDGE('',*,*,#44076,.T.);
#59110=ORIENTED_EDGE('',*,*,#44077,.T.);
#59111=ORIENTED_EDGE('',*,*,#44078,.F.);
#59112=ORIENTED_EDGE('',*,*,#44079,.T.);
#59113=ORIENTED_EDGE('',*,*,#44065,.F.);
#59114=ORIENTED_EDGE('',*,*,#44080,.F.);
#59115=ORIENTED_EDGE('',*,*,#44081,.T.);
#59116=ORIENTED_EDGE('',*,*,#44082,.F.);
#59117=ORIENTED_EDGE('',*,*,#44077,.F.);
#59118=ORIENTED_EDGE('',*,*,#44083,.F.);
#59119=ORIENTED_EDGE('',*,*,#44084,.T.);
#59120=ORIENTED_EDGE('',*,*,#44085,.F.);
#59121=ORIENTED_EDGE('',*,*,#44081,.F.);
#59122=ORIENTED_EDGE('',*,*,#44086,.F.);
#59123=ORIENTED_EDGE('',*,*,#44087,.T.);
#59124=ORIENTED_EDGE('',*,*,#44088,.F.);
#59125=ORIENTED_EDGE('',*,*,#44084,.F.);
#59126=ORIENTED_EDGE('',*,*,#44089,.F.);
#59127=ORIENTED_EDGE('',*,*,#44090,.T.);
#59128=ORIENTED_EDGE('',*,*,#44091,.F.);
#59129=ORIENTED_EDGE('',*,*,#44087,.F.);
#59130=ORIENTED_EDGE('',*,*,#44092,.T.);
#59131=ORIENTED_EDGE('',*,*,#44093,.T.);
#59132=ORIENTED_EDGE('',*,*,#44094,.T.);
#59133=ORIENTED_EDGE('',*,*,#44093,.F.);
#59134=ORIENTED_EDGE('',*,*,#44095,.T.);
#59135=ORIENTED_EDGE('',*,*,#44096,.F.);
#59136=ORIENTED_EDGE('',*,*,#44090,.F.);
#59137=ORIENTED_EDGE('',*,*,#44097,.F.);
#59138=ORIENTED_EDGE('',*,*,#44098,.T.);
#59139=ORIENTED_EDGE('',*,*,#44099,.F.);
#59140=ORIENTED_EDGE('',*,*,#44056,.F.);
#59141=ORIENTED_EDGE('',*,*,#44100,.F.);
#59142=ORIENTED_EDGE('',*,*,#44101,.T.);
#59143=ORIENTED_EDGE('',*,*,#44102,.F.);
#59144=ORIENTED_EDGE('',*,*,#44060,.F.);
#59145=ORIENTED_EDGE('',*,*,#44103,.F.);
#59146=ORIENTED_EDGE('',*,*,#44104,.T.);
#59147=ORIENTED_EDGE('',*,*,#44105,.F.);
#59148=ORIENTED_EDGE('',*,*,#44063,.F.);
#59149=ORIENTED_EDGE('',*,*,#44106,.F.);
#59150=ORIENTED_EDGE('',*,*,#44107,.T.);
#59151=ORIENTED_EDGE('',*,*,#44094,.F.);
#59152=ORIENTED_EDGE('',*,*,#44107,.F.);
#59153=ORIENTED_EDGE('',*,*,#44108,.T.);
#59154=ORIENTED_EDGE('',*,*,#44109,.T.);
#59155=ORIENTED_EDGE('',*,*,#44108,.F.);
#59156=ORIENTED_EDGE('',*,*,#44109,.F.);
#59157=ORIENTED_EDGE('',*,*,#44064,.T.);
#59158=ORIENTED_EDGE('',*,*,#44085,.T.);
#59159=ORIENTED_EDGE('',*,*,#44088,.T.);
#59160=ORIENTED_EDGE('',*,*,#44091,.T.);
#59161=ORIENTED_EDGE('',*,*,#44096,.T.);
#59162=ORIENTED_EDGE('',*,*,#44110,.T.);
#59163=ORIENTED_EDGE('',*,*,#44078,.T.);
#59164=ORIENTED_EDGE('',*,*,#44082,.T.);
#59165=ORIENTED_EDGE('',*,*,#44044,.T.);
#59166=ORIENTED_EDGE('',*,*,#44035,.T.);
#59167=ORIENTED_EDGE('',*,*,#44067,.F.);
#59168=ORIENTED_EDGE('',*,*,#44111,.T.);
#59169=ORIENTED_EDGE('',*,*,#44106,.T.);
#59170=ORIENTED_EDGE('',*,*,#44062,.T.);
#59171=ORIENTED_EDGE('',*,*,#44053,.T.);
#59172=ORIENTED_EDGE('',*,*,#44110,.F.);
#59173=ORIENTED_EDGE('',*,*,#44095,.F.);
#59174=ORIENTED_EDGE('',*,*,#44092,.F.);
#59175=ORIENTED_EDGE('',*,*,#44111,.F.);
#59176=ORIENTED_EDGE('',*,*,#44066,.F.);
#59177=ORIENTED_EDGE('',*,*,#44079,.F.);
#59178=ORIENTED_EDGE('',*,*,#44039,.T.);
#59179=ORIENTED_EDGE('',*,*,#44048,.T.);
#59180=ORIENTED_EDGE('',*,*,#44057,.T.);
#59181=ORIENTED_EDGE('',*,*,#44099,.T.);
#59182=ORIENTED_EDGE('',*,*,#44112,.T.);
#59183=ORIENTED_EDGE('',*,*,#44074,.T.);
#59184=ORIENTED_EDGE('',*,*,#44027,.T.);
#59185=ORIENTED_EDGE('',*,*,#44083,.T.);
#59186=ORIENTED_EDGE('',*,*,#44080,.T.);
#59187=ORIENTED_EDGE('',*,*,#44076,.F.);
#59188=ORIENTED_EDGE('',*,*,#44113,.T.);
#59189=ORIENTED_EDGE('',*,*,#44097,.T.);
#59190=ORIENTED_EDGE('',*,*,#44089,.T.);
#59191=ORIENTED_EDGE('',*,*,#44086,.T.);
#59192=ORIENTED_EDGE('',*,*,#44112,.F.);
#59193=ORIENTED_EDGE('',*,*,#44098,.F.);
#59194=ORIENTED_EDGE('',*,*,#44113,.F.);
#59195=ORIENTED_EDGE('',*,*,#44075,.F.);
#59196=ORIENTED_EDGE('',*,*,#44041,.T.);
#59197=ORIENTED_EDGE('',*,*,#44031,.T.);
#59198=ORIENTED_EDGE('',*,*,#44070,.F.);
#59199=ORIENTED_EDGE('',*,*,#44114,.T.);
#59200=ORIENTED_EDGE('',*,*,#44103,.T.);
#59201=ORIENTED_EDGE('',*,*,#44059,.T.);
#59202=ORIENTED_EDGE('',*,*,#44050,.T.);
#59203=ORIENTED_EDGE('',*,*,#44043,.T.);
#59204=ORIENTED_EDGE('',*,*,#44052,.T.);
#59205=ORIENTED_EDGE('',*,*,#44061,.T.);
#59206=ORIENTED_EDGE('',*,*,#44105,.T.);
#59207=ORIENTED_EDGE('',*,*,#44115,.T.);
#59208=ORIENTED_EDGE('',*,*,#44068,.T.);
#59209=ORIENTED_EDGE('',*,*,#44033,.T.);
#59210=ORIENTED_EDGE('',*,*,#44115,.F.);
#59211=ORIENTED_EDGE('',*,*,#44104,.F.);
#59212=ORIENTED_EDGE('',*,*,#44114,.F.);
#59213=ORIENTED_EDGE('',*,*,#44069,.F.);
#59214=ORIENTED_EDGE('',*,*,#44037,.T.);
#59215=ORIENTED_EDGE('',*,*,#44025,.T.);
#59216=ORIENTED_EDGE('',*,*,#44073,.F.);
#59217=ORIENTED_EDGE('',*,*,#44116,.T.);
#59218=ORIENTED_EDGE('',*,*,#44100,.T.);
#59219=ORIENTED_EDGE('',*,*,#44055,.T.);
#59220=ORIENTED_EDGE('',*,*,#44046,.T.);
#59221=ORIENTED_EDGE('',*,*,#44040,.T.);
#59222=ORIENTED_EDGE('',*,*,#44049,.T.);
#59223=ORIENTED_EDGE('',*,*,#44058,.T.);
#59224=ORIENTED_EDGE('',*,*,#44102,.T.);
#59225=ORIENTED_EDGE('',*,*,#44117,.T.);
#59226=ORIENTED_EDGE('',*,*,#44071,.T.);
#59227=ORIENTED_EDGE('',*,*,#44029,.T.);
#59228=ORIENTED_EDGE('',*,*,#44117,.F.);
#59229=ORIENTED_EDGE('',*,*,#44101,.F.);
#59230=ORIENTED_EDGE('',*,*,#44116,.F.);
#59231=ORIENTED_EDGE('',*,*,#44072,.F.);
#59232=ORIENTED_EDGE('',*,*,#44118,.T.);
#59233=ORIENTED_EDGE('',*,*,#44119,.T.);
#59234=ORIENTED_EDGE('',*,*,#44120,.T.);
#59235=ORIENTED_EDGE('',*,*,#44121,.T.);
#59236=ORIENTED_EDGE('',*,*,#44121,.F.);
#59237=ORIENTED_EDGE('',*,*,#44122,.T.);
#59238=ORIENTED_EDGE('',*,*,#44123,.F.);
#59239=ORIENTED_EDGE('',*,*,#44124,.F.);
#59240=ORIENTED_EDGE('',*,*,#44120,.F.);
#59241=ORIENTED_EDGE('',*,*,#44125,.T.);
#59242=ORIENTED_EDGE('',*,*,#44126,.F.);
#59243=ORIENTED_EDGE('',*,*,#44127,.T.);
#59244=ORIENTED_EDGE('',*,*,#44128,.F.);
#59245=ORIENTED_EDGE('',*,*,#44129,.F.);
#59246=ORIENTED_EDGE('',*,*,#44130,.F.);
#59247=ORIENTED_EDGE('',*,*,#44131,.T.);
#59248=ORIENTED_EDGE('',*,*,#44132,.T.);
#59249=ORIENTED_EDGE('',*,*,#44133,.F.);
#59250=ORIENTED_EDGE('',*,*,#44134,.F.);
#59251=ORIENTED_EDGE('',*,*,#44122,.F.);
#59252=ORIENTED_EDGE('',*,*,#44135,.T.);
#59253=ORIENTED_EDGE('',*,*,#44123,.T.);
#59254=ORIENTED_EDGE('',*,*,#44134,.T.);
#59255=ORIENTED_EDGE('',*,*,#44136,.T.);
#59256=ORIENTED_EDGE('',*,*,#44136,.F.);
#59257=ORIENTED_EDGE('',*,*,#44133,.T.);
#59258=ORIENTED_EDGE('',*,*,#44137,.T.);
#59259=ORIENTED_EDGE('',*,*,#44138,.F.);
#59260=ORIENTED_EDGE('',*,*,#44139,.T.);
#59261=ORIENTED_EDGE('',*,*,#44140,.T.);
#59262=ORIENTED_EDGE('',*,*,#44126,.T.);
#59263=ORIENTED_EDGE('',*,*,#44141,.T.);
#59264=ORIENTED_EDGE('',*,*,#44119,.F.);
#59265=ORIENTED_EDGE('',*,*,#44142,.F.);
#59266=ORIENTED_EDGE('',*,*,#44141,.F.);
#59267=ORIENTED_EDGE('',*,*,#44125,.F.);
#59268=ORIENTED_EDGE('',*,*,#44143,.T.);
#59269=ORIENTED_EDGE('',*,*,#44144,.T.);
#59270=ORIENTED_EDGE('',*,*,#44128,.T.);
#59271=ORIENTED_EDGE('',*,*,#44145,.T.);
#59272=ORIENTED_EDGE('',*,*,#44144,.F.);
#59273=ORIENTED_EDGE('',*,*,#44146,.F.);
#59274=ORIENTED_EDGE('',*,*,#44147,.F.);
#59275=ORIENTED_EDGE('',*,*,#44129,.T.);
#59276=ORIENTED_EDGE('',*,*,#44131,.F.);
#59277=ORIENTED_EDGE('',*,*,#44148,.T.);
#59278=ORIENTED_EDGE('',*,*,#44149,.F.);
#59279=ORIENTED_EDGE('',*,*,#44150,.F.);
#59280=ORIENTED_EDGE('',*,*,#44151,.T.);
#59281=ORIENTED_EDGE('',*,*,#44152,.T.);
#59282=ORIENTED_EDGE('',*,*,#44153,.T.);
#59283=ORIENTED_EDGE('',*,*,#44149,.T.);
#59284=ORIENTED_EDGE('',*,*,#44154,.F.);
#59285=ORIENTED_EDGE('',*,*,#44155,.F.);
#59286=ORIENTED_EDGE('',*,*,#44156,.F.);
#59287=ORIENTED_EDGE('',*,*,#44152,.F.);
#59288=ORIENTED_EDGE('',*,*,#44156,.T.);
#59289=ORIENTED_EDGE('',*,*,#44157,.F.);
#59290=ORIENTED_EDGE('',*,*,#44137,.F.);
#59291=ORIENTED_EDGE('',*,*,#44132,.F.);
#59292=ORIENTED_EDGE('',*,*,#44150,.T.);
#59293=ORIENTED_EDGE('',*,*,#44153,.F.);
#59294=ORIENTED_EDGE('',*,*,#44140,.F.);
#59295=ORIENTED_EDGE('',*,*,#44158,.F.);
#59296=ORIENTED_EDGE('',*,*,#44145,.F.);
#59297=ORIENTED_EDGE('',*,*,#44127,.F.);
#59298=ORIENTED_EDGE('',*,*,#44130,.T.);
#59299=ORIENTED_EDGE('',*,*,#44147,.T.);
#59300=ORIENTED_EDGE('',*,*,#44159,.F.);
#59301=ORIENTED_EDGE('',*,*,#44154,.T.);
#59302=ORIENTED_EDGE('',*,*,#44151,.F.);
#59303=ORIENTED_EDGE('',*,*,#44148,.F.);
#59304=ORIENTED_EDGE('',*,*,#44118,.F.);
#59305=ORIENTED_EDGE('',*,*,#44124,.T.);
#59306=ORIENTED_EDGE('',*,*,#44135,.F.);
#59307=ORIENTED_EDGE('',*,*,#44138,.T.);
#59308=ORIENTED_EDGE('',*,*,#44157,.T.);
#59309=ORIENTED_EDGE('',*,*,#44155,.T.);
#59310=ORIENTED_EDGE('',*,*,#44159,.T.);
#59311=ORIENTED_EDGE('',*,*,#44146,.T.);
#59312=ORIENTED_EDGE('',*,*,#44143,.F.);
#59313=ORIENTED_EDGE('',*,*,#44158,.T.);
#59314=ORIENTED_EDGE('',*,*,#44139,.F.);
#59315=ORIENTED_EDGE('',*,*,#44142,.T.);
#87120=CYLINDRICAL_SURFACE('',#95271,2.);
#87121=CYLINDRICAL_SURFACE('',#95287,3.);
#87122=CYLINDRICAL_SURFACE('',#95296,5.);
#87123=CYLINDRICAL_SURFACE('',#95311,0.4);
#87124=CYLINDRICAL_SURFACE('',#95322,0.4);
#87125=CYLINDRICAL_SURFACE('',#95324,4.75);
#87126=CYLINDRICAL_SURFACE('',#95326,0.4);
#87127=CYLINDRICAL_SURFACE('',#95328,2.9);
#87128=CYLINDRICAL_SURFACE('',#95330,0.4);
#87129=CYLINDRICAL_SURFACE('',#95332,4.75);
#89000=ADVANCED_FACE('',(#6536),#5321,.T.);
#89001=ADVANCED_FACE('',(#6537),#5322,.T.);
#89002=ADVANCED_FACE('',(#6538),#5323,.T.);
#89003=ADVANCED_FACE('',(#6539),#4664,.T.);
#89004=ADVANCED_FACE('',(#6540),#4665,.T.);
#89005=ADVANCED_FACE('',(#6541),#4666,.T.);
#89006=ADVANCED_FACE('',(#6542),#4667,.T.);
#89007=ADVANCED_FACE('',(#6543),#4668,.T.);
#89008=ADVANCED_FACE('',(#6544),#4669,.T.);
#89009=ADVANCED_FACE('',(#6545),#5324,.T.);
#89010=ADVANCED_FACE('',(#6546),#5325,.T.);
#89011=ADVANCED_FACE('',(#6547),#5326,.T.);
#89012=ADVANCED_FACE('',(#6548),#87120,.F.);
#89013=ADVANCED_FACE('',(#6549),#5327,.T.);
#89014=ADVANCED_FACE('',(#6550),#4670,.T.);
#89015=ADVANCED_FACE('',(#6551),#4671,.T.);
#89016=ADVANCED_FACE('',(#6552),#5328,.T.);
#89017=ADVANCED_FACE('',(#6553),#87121,.T.);
#89018=ADVANCED_FACE('',(#6554,#5124),#5329,.T.);
#89019=ADVANCED_FACE('',(#6555),#87122,.T.);
#89020=ADVANCED_FACE('',(#6556,#5125),#5330,.T.);
#89021=ADVANCED_FACE('',(#6557),#5331,.F.);
#89022=ADVANCED_FACE('',(#6558),#5332,.F.);
#89023=ADVANCED_FACE('',(#6559),#5333,.T.);
#89024=ADVANCED_FACE('',(#6560),#5334,.F.);
#89025=ADVANCED_FACE('',(#6561),#5335,.F.);
#89026=ADVANCED_FACE('',(#6562),#5336,.T.);
#89027=ADVANCED_FACE('',(#6563),#5337,.F.);
#89028=ADVANCED_FACE('',(#6564),#5338,.F.);
#89029=ADVANCED_FACE('',(#6565),#5339,.T.);
#89030=ADVANCED_FACE('',(#6566),#5340,.F.);
#89031=ADVANCED_FACE('',(#6567),#5341,.F.);
#89032=ADVANCED_FACE('',(#6568),#5342,.T.);
#89033=ADVANCED_FACE('',(#6569),#87123,.T.);
#89034=ADVANCED_FACE('',(#6570),#5343,.T.);
#89035=ADVANCED_FACE('',(#6571),#5344,.F.);
#89036=ADVANCED_FACE('',(#6572),#87124,.T.);
#89037=ADVANCED_FACE('',(#6573),#87125,.T.);
#89038=ADVANCED_FACE('',(#6574),#87126,.T.);
#89039=ADVANCED_FACE('',(#6575),#87127,.F.);
#89040=ADVANCED_FACE('',(#6576),#87128,.T.);
#89041=ADVANCED_FACE('',(#6577),#87129,.T.);
#89042=ADVANCED_FACE('',(#6578),#5345,.T.);
#89043=ADVANCED_FACE('',(#6579),#5346,.T.);
#89044=ADVANCED_FACE('',(#6580),#5347,.T.);
#89045=ADVANCED_FACE('',(#6581),#5348,.T.);
#89046=ADVANCED_FACE('',(#6582),#5349,.T.);
#89047=ADVANCED_FACE('',(#6583),#5350,.T.);
#89048=ADVANCED_FACE('',(#6584),#5351,.T.);
#94624=CLOSED_SHELL('',(#89000,#89001,#89002,#89003,#89004,#89005,#89006,
#89007,#89008,#89009,#89010,#89011,#89012,#89013,#89014,#89015,#89016,#89017,
#89018,#89019,#89020,#89021,#89022,#89023,#89024,#89025,#89026,#89027,#89028,
#89029,#89030,#89031,#89032));
#94625=CLOSED_SHELL('',(#89033,#89034,#89035,#89036,#89037,#89038,#89039,
#89040,#89041,#89042,#89043,#89044,#89045,#89046,#89047,#89048));
#95243=AXIS2_PLACEMENT_3D('',#138408,#106475,#106476);
#95244=AXIS2_PLACEMENT_3D('',#138409,#106477,#106478);
#95245=AXIS2_PLACEMENT_3D('',#138414,#106480,#106481);
#95246=AXIS2_PLACEMENT_3D('',#138417,#106483,#106484);
#95247=AXIS2_PLACEMENT_3D('',#138418,#106485,#106486);
#95248=AXIS2_PLACEMENT_3D('',#138423,#106488,#106489);
#95249=AXIS2_PLACEMENT_3D('',#138426,#106491,#106492);
#95250=AXIS2_PLACEMENT_3D('',#138427,#106493,#106494);
#95251=AXIS2_PLACEMENT_3D('',#138432,#106496,#106497);
#95252=AXIS2_PLACEMENT_3D('',#138435,#106499,#106500);
#95253=AXIS2_PLACEMENT_3D('',#138436,#106501,#106502);
#95254=AXIS2_PLACEMENT_3D('',#138442,#106503,#106504);
#95255=AXIS2_PLACEMENT_3D('',#138446,#106505,#106506);
#95256=AXIS2_PLACEMENT_3D('',#138455,#106507,#106508);
#95257=AXIS2_PLACEMENT_3D('',#138456,#106509,#106510);
#95258=AXIS2_PLACEMENT_3D('',#138465,#106511,#106512);
#95259=AXIS2_PLACEMENT_3D('',#138466,#106513,#106514);
#95260=AXIS2_PLACEMENT_3D('',#138472,#106515,#106516);
#95261=AXIS2_PLACEMENT_3D('',#138476,#106517,#106518);
#95262=AXIS2_PLACEMENT_3D('',#138485,#106519,#106520);
#95263=AXIS2_PLACEMENT_3D('',#138486,#106521,#106522);
#95264=AXIS2_PLACEMENT_3D('',#138495,#106523,#106524);
#95265=AXIS2_PLACEMENT_3D('',#138496,#106525,#106526);
#95266=AXIS2_PLACEMENT_3D('',#138500,#106528,#106529);
#95267=AXIS2_PLACEMENT_3D('',#138502,#106531,#106532);
#95268=AXIS2_PLACEMENT_3D('',#138507,#106535,#106536);
#95269=AXIS2_PLACEMENT_3D('',#138508,#106537,#106538);
#95270=AXIS2_PLACEMENT_3D('',#138513,#106541,#106542);
#95271=AXIS2_PLACEMENT_3D('',#138514,#106543,#106544);
#95272=AXIS2_PLACEMENT_3D('',#138516,#106545,#106546);
#95273=AXIS2_PLACEMENT_3D('',#138520,#106548,#106549);
#95274=AXIS2_PLACEMENT_3D('',#138525,#106552,#106553);
#95275=AXIS2_PLACEMENT_3D('',#138530,#106556,#106557);
#95276=AXIS2_PLACEMENT_3D('',#138535,#106560,#106561);
#95277=AXIS2_PLACEMENT_3D('',#138539,#106563,#106564);
#95278=AXIS2_PLACEMENT_3D('',#138542,#106566,#106567);
#95279=AXIS2_PLACEMENT_3D('',#138543,#106568,#106569);
#95280=AXIS2_PLACEMENT_3D('',#138547,#106571,#106572);
#95281=AXIS2_PLACEMENT_3D('',#138549,#106574,#106575);
#95282=AXIS2_PLACEMENT_3D('',#138555,#106576,#106577);
#95283=AXIS2_PLACEMENT_3D('',#138559,#106578,#106579);
#95284=AXIS2_PLACEMENT_3D('',#138565,#106580,#106581);
#95285=AXIS2_PLACEMENT_3D('',#138569,#106582,#106583);
#95286=AXIS2_PLACEMENT_3D('',#138573,#106585,#106586);
#95287=AXIS2_PLACEMENT_3D('',#138575,#106588,#106589);
#95288=AXIS2_PLACEMENT_3D('',#138578,#106590,#106591);
#95289=AXIS2_PLACEMENT_3D('',#138581,#106593,#106594);
#95290=AXIS2_PLACEMENT_3D('',#138583,#106595,#106596);
#95291=AXIS2_PLACEMENT_3D('',#138588,#106599,#106600);
#95292=AXIS2_PLACEMENT_3D('',#138593,#106603,#106604);
#95293=AXIS2_PLACEMENT_3D('',#138598,#106607,#106608);
#95294=AXIS2_PLACEMENT_3D('',#138601,#106611,#106612);
#95295=AXIS2_PLACEMENT_3D('',#138603,#106613,#106614);
#95296=AXIS2_PLACEMENT_3D('',#138604,#106615,#106616);
#95297=AXIS2_PLACEMENT_3D('',#138607,#106618,#106619);
#95298=AXIS2_PLACEMENT_3D('',#138608,#106620,#106621);
#95299=AXIS2_PLACEMENT_3D('',#138609,#106622,#106623);
#95300=AXIS2_PLACEMENT_3D('',#138611,#106625,#106626);
#95301=AXIS2_PLACEMENT_3D('',#138613,#106628,#106629);
#95302=AXIS2_PLACEMENT_3D('',#138614,#106630,#106631);
#95303=AXIS2_PLACEMENT_3D('',#138616,#106633,#106634);
#95304=AXIS2_PLACEMENT_3D('',#138618,#106636,#106637);
#95305=AXIS2_PLACEMENT_3D('',#138619,#106638,#106639);
#95306=AXIS2_PLACEMENT_3D('',#138621,#106641,#106642);
#95307=AXIS2_PLACEMENT_3D('',#138623,#106644,#106645);
#95308=AXIS2_PLACEMENT_3D('',#138624,#106646,#106647);
#95309=AXIS2_PLACEMENT_3D('',#138626,#106649,#106650);
#95310=AXIS2_PLACEMENT_3D('',#138628,#106652,#106653);
#95311=AXIS2_PLACEMENT_3D('',#138629,#106654,#106655);
#95312=AXIS2_PLACEMENT_3D('',#138632,#106656,#106657);
#95313=AXIS2_PLACEMENT_3D('',#138636,#106659,#106660);
#95314=AXIS2_PLACEMENT_3D('',#138638,#106662,#106663);
#95315=AXIS2_PLACEMENT_3D('',#138644,#106667,#106668);
#95316=AXIS2_PLACEMENT_3D('',#138646,#106669,#106670);
#95317=AXIS2_PLACEMENT_3D('',#138648,#106671,#106672);
#95318=AXIS2_PLACEMENT_3D('',#138652,#106674,#106675);
#95319=AXIS2_PLACEMENT_3D('',#138654,#106676,#106677);
#95320=AXIS2_PLACEMENT_3D('',#138662,#106681,#106682);
#95321=AXIS2_PLACEMENT_3D('',#138663,#106683,#106684);
#95322=AXIS2_PLACEMENT_3D('',#138664,#106685,#106686);
#95323=AXIS2_PLACEMENT_3D('',#138666,#106687,#106688);
#95324=AXIS2_PLACEMENT_3D('',#138668,#106690,#106691);
#95325=AXIS2_PLACEMENT_3D('',#138671,#106693,#106694);
#95326=AXIS2_PLACEMENT_3D('',#138672,#106695,#106696);
#95327=AXIS2_PLACEMENT_3D('',#138675,#106697,#106698);
#95328=AXIS2_PLACEMENT_3D('',#138678,#106701,#106702);
#95329=AXIS2_PLACEMENT_3D('',#138679,#106703,#106704);
#95330=AXIS2_PLACEMENT_3D('',#138680,#106705,#106706);
#95331=AXIS2_PLACEMENT_3D('',#138683,#106707,#106708);
#95332=AXIS2_PLACEMENT_3D('',#138686,#106711,#106712);
#95333=AXIS2_PLACEMENT_3D('',#138688,#106713,#106714);
#95334=AXIS2_PLACEMENT_3D('',#138690,#106716,#106717);
#95335=AXIS2_PLACEMENT_3D('',#138696,#106721,#106722);
#95336=AXIS2_PLACEMENT_3D('',#138702,#106726,#106727);
#95337=AXIS2_PLACEMENT_3D('',#138708,#106731,#106732);
#95338=AXIS2_PLACEMENT_3D('',#138710,#106734,#106735);
#95339=AXIS2_PLACEMENT_3D('',#138712,#106737,#106738);
#95340=AXIS2_PLACEMENT_3D('',#138714,#106740,#106741);
#106475=DIRECTION('axis',(0.,0.,1.));
#106476=DIRECTION('refdir',(1.,0.,0.));
#106477=DIRECTION('center_axis',(0.,0.,-1.));
#106478=DIRECTION('ref_axis',(-1.,0.,0.));
#106479=DIRECTION('',(1.,-1.05190123196885E-16,0.));
#106480=DIRECTION('center_axis',(0.,0.,-1.));
#106481=DIRECTION('ref_axis',(-1.,0.,0.));
#106482=DIRECTION('',(1.75316871994808E-16,1.,0.));
#106483=DIRECTION('center_axis',(0.,0.,-1.));
#106484=DIRECTION('ref_axis',(-1.,0.,0.));
#106485=DIRECTION('center_axis',(0.,0.,-1.));
#106486=DIRECTION('ref_axis',(-1.,0.,0.));
#106487=DIRECTION('',(-1.,1.75316871994808E-16,0.));
#106488=DIRECTION('center_axis',(0.,0.,-1.));
#106489=DIRECTION('ref_axis',(-1.,0.,0.));
#106490=DIRECTION('',(1.05190123196885E-16,1.,0.));
#106491=DIRECTION('center_axis',(0.,0.,-1.));
#106492=DIRECTION('ref_axis',(-1.,0.,0.));
#106493=DIRECTION('center_axis',(0.,0.,-1.));
#106494=DIRECTION('ref_axis',(-1.,0.,0.));
#106495=DIRECTION('',(-1.75316871994808E-16,-1.,0.));
#106496=DIRECTION('center_axis',(0.,0.,-1.));
#106497=DIRECTION('ref_axis',(-1.,0.,0.));
#106498=DIRECTION('',(-1.,1.05190123196885E-16,0.));
#106499=DIRECTION('center_axis',(0.,0.,-1.));
#106500=DIRECTION('ref_axis',(-1.,0.,0.));
#106501=DIRECTION('center_axis',(0.,0.,1.));
#106502=DIRECTION('ref_axis',(1.,0.,0.));
#106503=DIRECTION('center_axis',(0.,0.,-1.));
#106504=DIRECTION('ref_axis',(-1.,0.,0.));
#106505=DIRECTION('center_axis',(0.,0.,1.));
#106506=DIRECTION('ref_axis',(1.,0.,0.));
#106507=DIRECTION('center_axis',(0.,0.,-1.));
#106508=DIRECTION('ref_axis',(-1.,0.,0.));
#106509=DIRECTION('center_axis',(0.,0.,1.));
#106510=DIRECTION('ref_axis',(1.,0.,0.));
#106511=DIRECTION('center_axis',(0.,0.,-1.));
#106512=DIRECTION('ref_axis',(-1.,0.,0.));
#106513=DIRECTION('center_axis',(0.,0.,-1.));
#106514=DIRECTION('ref_axis',(-1.,0.,0.));
#106515=DIRECTION('center_axis',(0.,0.,-1.));
#106516=DIRECTION('ref_axis',(-1.,0.,0.));
#106517=DIRECTION('center_axis',(0.,0.,-1.));
#106518=DIRECTION('ref_axis',(-1.,0.,0.));
#106519=DIRECTION('center_axis',(0.,0.,-1.));
#106520=DIRECTION('ref_axis',(-1.,0.,0.));
#106521=DIRECTION('center_axis',(0.,0.,-1.));
#106522=DIRECTION('ref_axis',(-1.,0.,0.));
#106523=DIRECTION('center_axis',(0.,0.,-1.));
#106524=DIRECTION('ref_axis',(-1.,0.,0.));
#106525=DIRECTION('center_axis',(0.,0.,1.));
#106526=DIRECTION('ref_axis',(1.,0.,0.));
#106527=DIRECTION('',(-1.,1.05190123196885E-16,0.));
#106528=DIRECTION('center_axis',(0.,0.,-1.));
#106529=DIRECTION('ref_axis',(-1.,0.,0.));
#106530=DIRECTION('',(-1.75316871994808E-16,-1.,0.));
#106531=DIRECTION('center_axis',(0.,0.,1.));
#106532=DIRECTION('ref_axis',(1.,0.,0.));
#106533=DIRECTION('',(1.,-1.75316871994808E-16,0.));
#106534=DIRECTION('',(-1.05190123196885E-16,-1.,0.));
#106535=DIRECTION('center_axis',(0.,0.,-1.));
#106536=DIRECTION('ref_axis',(-1.,0.,0.));
#106537=DIRECTION('center_axis',(0.,0.,1.));
#106538=DIRECTION('ref_axis',(1.,0.,0.));
#106539=DIRECTION('',(1.75316871994808E-16,1.,0.));
#106540=DIRECTION('',(1.,-1.05190123196885E-16,0.));
#106541=DIRECTION('center_axis',(0.,0.,-1.));
#106542=DIRECTION('ref_axis',(-1.,0.,0.));
#106543=DIRECTION('center_axis',(0.,0.,-1.));
#106544=DIRECTION('ref_axis',(-1.,0.,0.));
#106545=DIRECTION('center_axis',(0.,0.,-1.));
#106546=DIRECTION('ref_axis',(-1.,0.,0.));
#106547=DIRECTION('',(0.,0.,-1.));
#106548=DIRECTION('center_axis',(0.,0.,-1.));
#106549=DIRECTION('ref_axis',(-1.,0.,0.));
#106550=DIRECTION('',(0.,0.,-1.));
#106551=DIRECTION('',(0.,0.,-1.));
#106552=DIRECTION('center_axis',(0.,0.,-1.));
#106553=DIRECTION('ref_axis',(-1.,0.,0.));
#106554=DIRECTION('',(0.,0.,-1.));
#106555=DIRECTION('',(0.,0.,-1.));
#106556=DIRECTION('center_axis',(0.,0.,-1.));
#106557=DIRECTION('ref_axis',(-1.,0.,0.));
#106558=DIRECTION('',(0.,0.,-1.));
#106559=DIRECTION('',(0.,0.,-1.));
#106560=DIRECTION('center_axis',(0.,0.,-1.));
#106561=DIRECTION('ref_axis',(-1.,0.,0.));
#106562=DIRECTION('',(0.,0.,-1.));
#106563=DIRECTION('center_axis',(0.,0.,-1.));
#106564=DIRECTION('ref_axis',(-1.,0.,0.));
#106565=DIRECTION('',(0.,0.,-1.));
#106566=DIRECTION('center_axis',(0.,0.,-1.));
#106567=DIRECTION('ref_axis',(-1.,0.,0.));
#106568=DIRECTION('center_axis',(0.,0.,-1.));
#106569=DIRECTION('ref_axis',(-1.,0.,0.));
#106570=DIRECTION('',(-1.05190123196885E-16,-1.,0.));
#106571=DIRECTION('center_axis',(0.,0.,-1.));
#106572=DIRECTION('ref_axis',(-1.,0.,0.));
#106573=DIRECTION('',(1.,-1.75316871994808E-16,0.));
#106574=DIRECTION('center_axis',(0.,0.,1.));
#106575=DIRECTION('ref_axis',(1.,0.,0.));
#106576=DIRECTION('center_axis',(0.,0.,-1.));
#106577=DIRECTION('ref_axis',(-1.,0.,0.));
#106578=DIRECTION('center_axis',(0.,0.,-1.));
#106579=DIRECTION('ref_axis',(-1.,0.,0.));
#106580=DIRECTION('center_axis',(0.,0.,-1.));
#106581=DIRECTION('ref_axis',(-1.,0.,0.));
#106582=DIRECTION('center_axis',(0.,0.,1.));
#106583=DIRECTION('ref_axis',(1.,0.,0.));
#106584=DIRECTION('',(1.05190123196885E-16,1.,0.));
#106585=DIRECTION('center_axis',(0.,0.,-1.));
#106586=DIRECTION('ref_axis',(-1.,0.,0.));
#106587=DIRECTION('',(-1.,1.75316871994808E-16,0.));
#106588=DIRECTION('center_axis',(0.,0.,-1.));
#106589=DIRECTION('ref_axis',(-1.,0.,0.));
#106590=DIRECTION('center_axis',(0.,0.,-1.));
#106591=DIRECTION('ref_axis',(-1.,0.,0.));
#106592=DIRECTION('',(0.,0.,1.));
#106593=DIRECTION('center_axis',(0.,0.,-1.));
#106594=DIRECTION('ref_axis',(-1.,0.,0.));
#106595=DIRECTION('center_axis',(0.,0.,-1.));
#106596=DIRECTION('ref_axis',(-1.,0.,0.));
#106597=DIRECTION('',(0.,0.,-1.));
#106598=DIRECTION('',(0.,0.,-1.));
#106599=DIRECTION('center_axis',(0.,0.,-1.));
#106600=DIRECTION('ref_axis',(-1.,0.,0.));
#106601=DIRECTION('',(0.,0.,-1.));
#106602=DIRECTION('',(0.,0.,-1.));
#106603=DIRECTION('center_axis',(0.,0.,-1.));
#106604=DIRECTION('ref_axis',(-1.,0.,0.));
#106605=DIRECTION('',(0.,0.,-1.));
#106606=DIRECTION('',(0.,0.,-1.));
#106607=DIRECTION('center_axis',(0.,0.,-1.));
#106608=DIRECTION('ref_axis',(-1.,0.,0.));
#106609=DIRECTION('',(0.,0.,-1.));
#106610=DIRECTION('',(0.,0.,-1.));
#106611=DIRECTION('center_axis',(0.,0.,-1.));
#106612=DIRECTION('ref_axis',(-1.,0.,0.));
#106613=DIRECTION('center_axis',(0.,0.,-1.));
#106614=DIRECTION('ref_axis',(-1.,0.,0.));
#106615=DIRECTION('center_axis',(0.,0.,-1.));
#106616=DIRECTION('ref_axis',(-1.,0.,0.));
#106617=DIRECTION('',(0.,0.,1.));
#106618=DIRECTION('center_axis',(0.,0.,-1.));
#106619=DIRECTION('ref_axis',(-1.,0.,0.));
#106620=DIRECTION('center_axis',(0.,0.,1.));
#106621=DIRECTION('ref_axis',(1.,0.,0.));
#106622=DIRECTION('center_axis',(1.75316871994808E-16,1.,0.));
#106623=DIRECTION('ref_axis',(-1.,1.75316871994808E-16,0.));
#106624=DIRECTION('',(1.,-1.75316871994808E-16,0.));
#106625=DIRECTION('center_axis',(-1.05190123196885E-16,-1.,0.));
#106626=DIRECTION('ref_axis',(1.,-1.05190123196885E-16,0.));
#106627=DIRECTION('',(-1.,1.05190123196885E-16,0.));
#106628=DIRECTION('center_axis',(0.,0.,-1.));
#106629=DIRECTION('ref_axis',(-1.,0.,0.));
#106630=DIRECTION('center_axis',(-1.,1.75316871994808E-16,0.));
#106631=DIRECTION('ref_axis',(-1.75316871994808E-16,-1.,0.));
#106632=DIRECTION('',(1.75316871994808E-16,1.,0.));
#106633=DIRECTION('center_axis',(1.,-1.05190123196885E-16,0.));
#106634=DIRECTION('ref_axis',(1.05190123196885E-16,1.,0.));
#106635=DIRECTION('',(-1.05190123196885E-16,-1.,0.));
#106636=DIRECTION('center_axis',(0.,0.,-1.));
#106637=DIRECTION('ref_axis',(-1.,0.,0.));
#106638=DIRECTION('center_axis',(-1.,1.05190123196885E-16,0.));
#106639=DIRECTION('ref_axis',(-1.05190123196885E-16,-1.,0.));
#106640=DIRECTION('',(1.05190123196885E-16,1.,0.));
#106641=DIRECTION('center_axis',(1.,-1.75316871994808E-16,0.));
#106642=DIRECTION('ref_axis',(1.75316871994808E-16,1.,0.));
#106643=DIRECTION('',(-1.75316871994808E-16,-1.,0.));
#106644=DIRECTION('center_axis',(0.,0.,-1.));
#106645=DIRECTION('ref_axis',(-1.,0.,0.));
#106646=DIRECTION('center_axis',(1.05190123196885E-16,1.,0.));
#106647=DIRECTION('ref_axis',(-1.,1.05190123196885E-16,0.));
#106648=DIRECTION('',(1.,-1.05190123196885E-16,0.));
#106649=DIRECTION('center_axis',(-1.75316871994808E-16,-1.,0.));
#106650=DIRECTION('ref_axis',(1.,-1.75316871994808E-16,0.));
#106651=DIRECTION('',(-1.,1.75316871994808E-16,0.));
#106652=DIRECTION('center_axis',(0.,0.,-1.));
#106653=DIRECTION('ref_axis',(-1.,0.,0.));
#106654=DIRECTION('center_axis',(0.,0.,-1.));
#106655=DIRECTION('ref_axis',(-0.953462589245592,-0.301511344577763,0.));
#106656=DIRECTION('center_axis',(1.66533453693558E-16,-1.98164517174841E-27,
1.));
#106657=DIRECTION('ref_axis',(-0.953462589245592,-0.301511344577763,0.));
#106658=DIRECTION('',(0.,0.,1.));
#106659=DIRECTION('center_axis',(-1.66533453693558E-16,1.98164517174841E-27,
-1.));
#106660=DIRECTION('ref_axis',(-0.953462589245592,-0.301511344577763,0.));
#106661=DIRECTION('',(0.,0.,-1.));
#106662=DIRECTION('center_axis',(-1.,4.69089087030665E-43,0.));
#106663=DIRECTION('ref_axis',(4.69089087030665E-43,1.,1.98164517174841E-27));
#106664=DIRECTION('',(4.69089087030665E-43,1.,1.98164517174841E-27));
#106665=DIRECTION('',(0.,0.,1.));
#106666=DIRECTION('',(4.69089087030665E-43,1.,1.98164517174841E-27));
#106667=DIRECTION('center_axis',(-1.66533453693558E-16,1.98164517174841E-27,
-1.));
#106668=DIRECTION('ref_axis',(1.,-1.39078872584238E-43,-1.66533453693558E-16));
#106669=DIRECTION('center_axis',(-1.66533453693558E-16,1.98164517174841E-27,
-1.));
#106670=DIRECTION('ref_axis',(0.793103448275862,0.609086956298473,-1.32078256376442E-16));
#106671=DIRECTION('center_axis',(-1.66533453693558E-16,1.98164517174841E-27,
-1.));
#106672=DIRECTION('ref_axis',(0.953462589245592,-0.301511344577763,0.));
#106673=DIRECTION('',(4.69089087030665E-43,1.,1.98164517174841E-27));
#106674=DIRECTION('center_axis',(-1.66533453693558E-16,1.98164517174841E-27,
-1.));
#106675=DIRECTION('ref_axis',(0.435494170355695,0.900191550497007,0.));
#106676=DIRECTION('center_axis',(-1.66533453693558E-16,1.98164517174841E-27,
-1.));
#106677=DIRECTION('ref_axis',(-0.589473684210526,-0.807787580755776,9.81670884914437E-17));
#106678=DIRECTION('',(4.69089087030665E-43,1.,1.98164517174841E-27));
#106679=DIRECTION('',(1.,-1.39078872584238E-43,-1.66533453693558E-16));
#106680=DIRECTION('',(4.69089087030665E-43,1.,1.98164517174841E-27));
#106681=DIRECTION('center_axis',(-1.66533453693558E-16,1.98164517174841E-27,
-1.));
#106682=DIRECTION('ref_axis',(0.484210526315789,0.874951522202794,-8.06372512604098E-17));
#106683=DIRECTION('center_axis',(-1.66533453693558E-16,1.98164517174841E-27,
-1.));
#106684=DIRECTION('ref_axis',(-0.435494170355695,0.900191550497007,0.));
#106685=DIRECTION('center_axis',(0.,0.,-1.));
#106686=DIRECTION('ref_axis',(-0.435494170355695,0.900191550497007,0.));
#106687=DIRECTION('center_axis',(1.66533453693558E-16,-1.98164517174841E-27,
1.));
#106688=DIRECTION('ref_axis',(-0.435494170355695,0.900191550497007,0.));
#106689=DIRECTION('',(0.,0.,-1.));
#106690=DIRECTION('center_axis',(0.,0.,-1.));
#106691=DIRECTION('ref_axis',(0.484210526315789,0.874951522202794,0.));
#106692=DIRECTION('',(0.,0.,-1.));
#106693=DIRECTION('center_axis',(-1.66533453693558E-16,1.98164517174841E-27,
-1.));
#106694=DIRECTION('ref_axis',(0.484210526315789,0.874951522202794,-8.06372512604098E-17));
#106695=DIRECTION('center_axis',(0.,0.,-1.));
#106696=DIRECTION('ref_axis',(0.953462589245592,-0.301511344577763,0.));
#106697=DIRECTION('center_axis',(1.66533453693558E-16,-1.98164517174841E-27,
1.));
#106698=DIRECTION('ref_axis',(0.953462589245592,-0.301511344577763,0.));
#106699=DIRECTION('',(0.,0.,1.));
#106700=DIRECTION('',(0.,0.,-1.));
#106701=DIRECTION('center_axis',(0.,0.,-1.));
#106702=DIRECTION('ref_axis',(1.91417762866406E-16,-1.,0.));
#106703=DIRECTION('center_axis',(1.66533453693558E-16,-1.98164517174841E-27,
1.));
#106704=DIRECTION('ref_axis',(0.793103448275862,0.609086956298473,-1.32078256376442E-16));
#106705=DIRECTION('center_axis',(0.,0.,-1.));
#106706=DIRECTION('ref_axis',(0.435494170355695,0.900191550497007,0.));
#106707=DIRECTION('center_axis',(1.66533453693558E-16,-1.98164517174841E-27,
1.));
#106708=DIRECTION('ref_axis',(0.435494170355695,0.900191550497007,0.));
#106709=DIRECTION('',(0.,0.,1.));
#106710=DIRECTION('',(0.,0.,-1.));
#106711=DIRECTION('center_axis',(0.,0.,-1.));
#106712=DIRECTION('ref_axis',(-0.589473684210526,-0.807787580755776,0.));
#106713=DIRECTION('center_axis',(-1.66533453693558E-16,1.98164517174841E-27,
-1.));
#106714=DIRECTION('ref_axis',(-0.589473684210526,-0.807787580755776,9.81670884914437E-17));
#106715=DIRECTION('',(0.,0.,-1.));
#106716=DIRECTION('center_axis',(1.39078872584238E-43,1.,-4.28912684949805E-59));
#106717=DIRECTION('ref_axis',(-1.,1.39078872584238E-43,1.66533453693558E-16));
#106718=DIRECTION('',(3.08395284618099E-16,0.,1.));
#106719=DIRECTION('',(-1.,1.39078872584238E-43,1.66533453693558E-16));
#106720=DIRECTION('',(3.08395284618099E-16,0.,1.));
#106721=DIRECTION('center_axis',(3.08395284618099E-16,0.,1.));
#106722=DIRECTION('ref_axis',(1.,0.,-3.08395284618099E-16));
#106723=DIRECTION('',(-4.69089087030665E-43,-1.,-1.98164517174841E-27));
#106724=DIRECTION('',(1.,-1.39078872584238E-43,-1.66533453693558E-16));
#106725=DIRECTION('',(4.69089087030665E-43,1.,1.98164517174841E-27));
#106726=DIRECTION('center_axis',(-1.39078872584238E-43,-1.,0.));
#106727=DIRECTION('ref_axis',(-1.,1.39078872584238E-43,1.66533453693558E-16));
#106728=DIRECTION('',(3.08395284618099E-16,0.,1.));
#106729=DIRECTION('',(-1.,1.39078872584238E-43,1.66533453693558E-16));
#106730=DIRECTION('',(0.,0.,-1.));
#106731=DIRECTION('center_axis',(1.,-4.69089087030665E-43,0.));
#106732=DIRECTION('ref_axis',(-4.69089087030665E-43,-1.,-1.98164517174841E-27));
#106733=DIRECTION('',(-4.69089087030665E-43,-1.,-1.98164517174841E-27));
#106734=DIRECTION('center_axis',(1.,-4.69089087030665E-43,0.));
#106735=DIRECTION('ref_axis',(-4.69089087030665E-43,-1.,-1.98164517174841E-27));
#106736=DIRECTION('',(-4.69089087030665E-43,-1.,-1.98164517174841E-27));
#106737=DIRECTION('center_axis',(-1.,4.69089087030665E-43,0.));
#106738=DIRECTION('ref_axis',(4.69089087030665E-43,1.,1.98164517174841E-27));
#106739=DIRECTION('',(4.69089087030665E-43,1.,1.98164517174841E-27));
#106740=DIRECTION('center_axis',(-1.66533453693558E-16,1.98164517174841E-27,
-1.));
#106741=DIRECTION('ref_axis',(1.,-1.39078872584238E-43,-1.66533453693558E-16));
#138408=CARTESIAN_POINT('',(0.,0.,0.));
#138409=CARTESIAN_POINT('Origin',(2.,0.,0.));
#138410=CARTESIAN_POINT('',(-3.44818792991333,0.6,0.));
#138411=CARTESIAN_POINT('',(-1.90787840283389,0.6,0.));
#138412=CARTESIAN_POINT('',(-5.,0.6,0.));
#138413=CARTESIAN_POINT('',(-0.599999999999999,3.44818792991333,0.));
#138414=CARTESIAN_POINT('Origin',(0.,0.,0.));
#138415=CARTESIAN_POINT('',(-0.6,1.90787840283389,0.));
#138416=CARTESIAN_POINT('',(-0.6,1.90787840283389,0.));
#138417=CARTESIAN_POINT('Origin',(0.,0.,0.));
#138418=CARTESIAN_POINT('Origin',(2.,0.,0.));
#138419=CARTESIAN_POINT('',(-1.90787840283389,-0.6,0.));
#138420=CARTESIAN_POINT('',(-3.44818792991333,-0.599999999999999,0.));
#138421=CARTESIAN_POINT('',(-1.90787840283389,-0.6,0.));
#138422=CARTESIAN_POINT('',(-0.6,-1.90787840283389,0.));
#138423=CARTESIAN_POINT('Origin',(0.,0.,0.));
#138424=CARTESIAN_POINT('',(-0.6,-3.44818792991333,0.));
#138425=CARTESIAN_POINT('',(-0.6,-5.,0.));
#138426=CARTESIAN_POINT('Origin',(0.,0.,0.));
#138427=CARTESIAN_POINT('Origin',(2.,0.,0.));
#138428=CARTESIAN_POINT('',(0.6,-1.90787840283389,0.));
#138429=CARTESIAN_POINT('',(0.599999999999999,-3.44818792991333,0.));
#138430=CARTESIAN_POINT('',(0.6,-1.90787840283389,0.));
#138431=CARTESIAN_POINT('',(1.90787840283389,-0.6,0.));
#138432=CARTESIAN_POINT('Origin',(0.,0.,0.));
#138433=CARTESIAN_POINT('',(3.44818792991333,-0.6,0.));
#138434=CARTESIAN_POINT('',(5.,-0.6,0.));
#138435=CARTESIAN_POINT('Origin',(0.,0.,0.));
#138436=CARTESIAN_POINT('Origin',(0.,0.,0.));
#138437=CARTESIAN_POINT('',(-3.95474398665704,0.6,1.5));
#138438=CARTESIAN_POINT('Ctrl Pts',(-3.95474398665705,0.6,1.49999999999998));
#138439=CARTESIAN_POINT('Ctrl Pts',(-3.68458075639299,0.6,0.698680192272979));
#138440=CARTESIAN_POINT('Ctrl Pts',(-3.44818792991332,0.6,-1.17676210180771E-13));
#138441=CARTESIAN_POINT('',(-0.599999999999999,3.95474398665704,1.5));
#138442=CARTESIAN_POINT('Origin',(0.,0.,1.5));
#138443=CARTESIAN_POINT('Ctrl Pts',(-0.6,3.4481879299133,-1.06445473175915E-13));
#138444=CARTESIAN_POINT('Ctrl Pts',(-0.6,3.68458075639367,0.698680192275089));
#138445=CARTESIAN_POINT('Ctrl Pts',(-0.6,3.95474398665703,1.49999999999999));
#138446=CARTESIAN_POINT('Origin',(0.,0.,0.));
#138447=CARTESIAN_POINT('',(-3.95474398665704,-0.599999999999999,1.5));
#138448=CARTESIAN_POINT('Ctrl Pts',(-3.4481879299133,-0.6,-1.05897632346403E-13));
#138449=CARTESIAN_POINT('Ctrl Pts',(-3.68458075639369,-0.6,0.698680192275146));
#138450=CARTESIAN_POINT('Ctrl Pts',(-3.95474398665703,-0.6,1.49999999999999));
#138451=CARTESIAN_POINT('',(-0.6,-3.95474398665704,1.5));
#138452=CARTESIAN_POINT('Ctrl Pts',(-0.6,-3.95474398665703,1.49999999999999));
#138453=CARTESIAN_POINT('Ctrl Pts',(-0.6,-3.68458075639366,0.698680192275045));
#138454=CARTESIAN_POINT('Ctrl Pts',(-0.6,-3.4481879299133,-1.08088995664484E-13));
#138455=CARTESIAN_POINT('Origin',(0.,0.,1.5));
#138456=CARTESIAN_POINT('Origin',(0.,0.,0.));
#138457=CARTESIAN_POINT('',(0.599999999999999,-3.95474398665704,1.5));
#138458=CARTESIAN_POINT('Ctrl Pts',(0.6,-3.4481879299133,-1.06609825424756E-13));
#138459=CARTESIAN_POINT('Ctrl Pts',(0.6,-3.6845807563937,0.698680192275154));
#138460=CARTESIAN_POINT('Ctrl Pts',(0.6,-3.95474398665703,1.49999999999999));
#138461=CARTESIAN_POINT('',(3.95474398665704,-0.6,1.5));
#138462=CARTESIAN_POINT('Ctrl Pts',(3.95474398665703,-0.6,1.49999999999999));
#138463=CARTESIAN_POINT('Ctrl Pts',(3.68458075639368,-0.6,0.698680192275095));
#138464=CARTESIAN_POINT('Ctrl Pts',(3.4481879299133,-0.6,-1.03267996364691E-13));
#138465=CARTESIAN_POINT('Origin',(0.,0.,1.5));
#138466=CARTESIAN_POINT('Origin',(0.,0.,1.5));
#138467=CARTESIAN_POINT('',(-3.44818792991333,0.6,2.3));
#138468=CARTESIAN_POINT('Ctrl Pts',(-3.44818792991347,0.6,2.29999999999978));
#138469=CARTESIAN_POINT('Ctrl Pts',(-3.68458075656704,0.6,1.92737056384667));
#138470=CARTESIAN_POINT('Ctrl Pts',(-3.95474398705481,0.6,1.49999999937077));
#138471=CARTESIAN_POINT('',(-0.599999999999999,3.44818792991333,2.3));
#138472=CARTESIAN_POINT('Origin',(0.,0.,2.3));
#138473=CARTESIAN_POINT('Ctrl Pts',(-0.6,3.95474398665704,1.5));
#138474=CARTESIAN_POINT('Ctrl Pts',(-0.6,3.68458075639373,1.92737056411986));
#138475=CARTESIAN_POINT('Ctrl Pts',(-0.6,3.44818792991333,2.3));
#138476=CARTESIAN_POINT('Origin',(0.,0.,1.5));
#138477=CARTESIAN_POINT('',(-3.44818792991333,-0.599999999999999,2.3));
#138478=CARTESIAN_POINT('Ctrl Pts',(-3.95474398665704,-0.6,1.5));
#138479=CARTESIAN_POINT('Ctrl Pts',(-3.68458075639373,-0.6,1.92737056411986));
#138480=CARTESIAN_POINT('Ctrl Pts',(-3.44818792991333,-0.6,2.3));
#138481=CARTESIAN_POINT('',(-0.6,-3.44818792991333,2.3));
#138482=CARTESIAN_POINT('Ctrl Pts',(-0.600000000000001,-3.44818792991364,
2.2999999999995));
#138483=CARTESIAN_POINT('Ctrl Pts',(-0.600000000000001,-3.68458075656713,
1.92737056384652));
#138484=CARTESIAN_POINT('Ctrl Pts',(-0.600000000000001,-3.95474398705479,
1.49999999937079));
#138485=CARTESIAN_POINT('Origin',(0.,0.,2.3));
#138486=CARTESIAN_POINT('Origin',(0.,0.,1.5));
#138487=CARTESIAN_POINT('',(0.6,-3.44818792991333,2.3));
#138488=CARTESIAN_POINT('Ctrl Pts',(0.6,-3.95474398665704,1.5));
#138489=CARTESIAN_POINT('Ctrl Pts',(0.6,-3.68458075639373,1.92737056411986));
#138490=CARTESIAN_POINT('Ctrl Pts',(0.6,-3.44818792991333,2.3));
#138491=CARTESIAN_POINT('',(3.44818792991333,-0.6,2.3));
#138492=CARTESIAN_POINT('Ctrl Pts',(3.44818792991362,-0.600000000000001,
2.29999999999954));
#138493=CARTESIAN_POINT('Ctrl Pts',(3.68458075656725,-0.600000000000001,
1.92737056384633));
#138494=CARTESIAN_POINT('Ctrl Pts',(3.95474398705511,-0.600000000000001,
1.49999999937029));
#138495=CARTESIAN_POINT('Origin',(0.,0.,2.3));
#138496=CARTESIAN_POINT('Origin',(3.49999999999999,0.,2.3));
#138497=CARTESIAN_POINT('',(-2.93938769133981,0.6,2.3));
#138498=CARTESIAN_POINT('',(3.49999999999999,0.599999999999999,2.3));
#138499=CARTESIAN_POINT('',(-0.6,2.93938769133981,2.3));
#138500=CARTESIAN_POINT('Origin',(0.,0.,2.3));
#138501=CARTESIAN_POINT('',(-0.599999999999999,7.18799175178712E-16,2.3));
#138502=CARTESIAN_POINT('Origin',(3.49999999999999,0.,2.3));
#138503=CARTESIAN_POINT('',(-2.93938769133981,-0.6,2.3));
#138504=CARTESIAN_POINT('',(3.49999999999999,-0.600000000000001,2.3));
#138505=CARTESIAN_POINT('',(-0.6,-2.93938769133981,2.3));
#138506=CARTESIAN_POINT('',(-0.599999999999999,4.31279505107227E-16,2.3));
#138507=CARTESIAN_POINT('Origin',(0.,0.,2.3));
#138508=CARTESIAN_POINT('Origin',(3.49999999999999,0.,2.3));
#138509=CARTESIAN_POINT('',(0.6,-2.93938769133981,2.3));
#138510=CARTESIAN_POINT('',(0.6,5.08418928784942E-16,2.3));
#138511=CARTESIAN_POINT('',(2.93938769133981,-0.6,2.3));
#138512=CARTESIAN_POINT('',(3.49999999999999,-0.6,2.3));
#138513=CARTESIAN_POINT('Origin',(0.,0.,2.3));
#138514=CARTESIAN_POINT('Origin',(0.,0.,0.));
#138515=CARTESIAN_POINT('',(2.,-2.44929359829471E-16,8.));
#138516=CARTESIAN_POINT('Origin',(0.,0.,8.));
#138517=CARTESIAN_POINT('',(2.,-2.44929359829471E-16,6.1));
#138518=CARTESIAN_POINT('',(2.,-2.44929359829471E-16,0.));
#138519=CARTESIAN_POINT('',(1.90787840283389,-0.6,6.1));
#138520=CARTESIAN_POINT('Origin',(0.,0.,6.1));
#138521=CARTESIAN_POINT('',(1.90787840283389,-0.6,6.1));
#138522=CARTESIAN_POINT('',(0.6,-1.90787840283389,6.1));
#138523=CARTESIAN_POINT('',(0.6,-1.90787840283389,6.1));
#138524=CARTESIAN_POINT('',(-0.6,-1.90787840283389,6.1));
#138525=CARTESIAN_POINT('Origin',(0.,0.,6.1));
#138526=CARTESIAN_POINT('',(-0.6,-1.90787840283389,6.1));
#138527=CARTESIAN_POINT('',(-1.90787840283389,-0.6,6.1));
#138528=CARTESIAN_POINT('',(-1.90787840283389,-0.6,6.1));
#138529=CARTESIAN_POINT('',(-1.90787840283389,0.6,6.1));
#138530=CARTESIAN_POINT('Origin',(0.,0.,6.1));
#138531=CARTESIAN_POINT('',(-1.90787840283389,0.6,6.1));
#138532=CARTESIAN_POINT('',(-0.6,1.90787840283389,6.1));
#138533=CARTESIAN_POINT('',(-0.6,1.90787840283389,6.1));
#138534=CARTESIAN_POINT('',(0.6,1.90787840283389,6.1));
#138535=CARTESIAN_POINT('Origin',(0.,0.,6.1));
#138536=CARTESIAN_POINT('',(0.6,1.90787840283389,0.));
#138537=CARTESIAN_POINT('',(0.6,1.90787840283389,6.1));
#138538=CARTESIAN_POINT('',(1.90787840283389,0.6,0.));
#138539=CARTESIAN_POINT('Origin',(0.,0.,0.));
#138540=CARTESIAN_POINT('',(1.90787840283389,0.6,6.1));
#138541=CARTESIAN_POINT('',(1.90787840283389,0.6,6.1));
#138542=CARTESIAN_POINT('Origin',(0.,0.,6.1));
#138543=CARTESIAN_POINT('Origin',(2.,0.,0.));
#138544=CARTESIAN_POINT('',(0.6,3.44818792991333,0.));
#138545=CARTESIAN_POINT('',(0.6,5.,0.));
#138546=CARTESIAN_POINT('',(3.44818792991333,0.599999999999999,0.));
#138547=CARTESIAN_POINT('Origin',(0.,0.,0.));
#138548=CARTESIAN_POINT('',(1.90787840283389,0.6,0.));
#138549=CARTESIAN_POINT('Origin',(0.,0.,0.));
#138550=CARTESIAN_POINT('',(0.6,3.95474398665704,1.5));
#138551=CARTESIAN_POINT('Ctrl Pts',(0.6,3.95474398665705,1.49999999999998));
#138552=CARTESIAN_POINT('Ctrl Pts',(0.6,3.68458075639299,0.698680192272979));
#138553=CARTESIAN_POINT('Ctrl Pts',(0.6,3.44818792991332,-1.17676210180771E-13));
#138554=CARTESIAN_POINT('',(3.95474398665704,0.599999999999999,1.5));
#138555=CARTESIAN_POINT('Origin',(0.,0.,1.5));
#138556=CARTESIAN_POINT('Ctrl Pts',(3.4481879299133,0.6,-1.06445473175915E-13));
#138557=CARTESIAN_POINT('Ctrl Pts',(3.68458075639367,0.6,0.698680192275089));
#138558=CARTESIAN_POINT('Ctrl Pts',(3.95474398665703,0.6,1.49999999999999));
#138559=CARTESIAN_POINT('Origin',(0.,0.,1.5));
#138560=CARTESIAN_POINT('',(0.6,3.44818792991333,2.3));
#138561=CARTESIAN_POINT('Ctrl Pts',(0.600000000000001,3.44818792991352,
2.2999999999997));
#138562=CARTESIAN_POINT('Ctrl Pts',(0.600000000000001,3.68458075656709,
1.92737056384658));
#138563=CARTESIAN_POINT('Ctrl Pts',(0.600000000000001,3.95474398705488,
1.49999999937066));
#138564=CARTESIAN_POINT('',(3.44818792991333,0.599999999999999,2.3));
#138565=CARTESIAN_POINT('Origin',(0.,0.,2.3));
#138566=CARTESIAN_POINT('Ctrl Pts',(3.95474398665705,0.599999999999999,
1.49999999999998));
#138567=CARTESIAN_POINT('Ctrl Pts',(3.68458075639374,0.599999999999999,
1.92737056411985));
#138568=CARTESIAN_POINT('Ctrl Pts',(3.44818792991334,0.599999999999999,
2.29999999999998));
#138569=CARTESIAN_POINT('Origin',(3.49999999999999,0.,2.3));
#138570=CARTESIAN_POINT('',(0.6,2.93938769133981,2.3));
#138571=CARTESIAN_POINT('',(0.6,3.05051357270965E-16,2.3));
#138572=CARTESIAN_POINT('',(2.93938769133981,0.6,2.3));
#138573=CARTESIAN_POINT('Origin',(0.,0.,2.3));
#138574=CARTESIAN_POINT('',(3.49999999999999,0.599999999999999,2.3));
#138575=CARTESIAN_POINT('Origin',(0.,0.,0.));
#138576=CARTESIAN_POINT('',(2.93938769133981,-0.6,6.1));
#138577=CARTESIAN_POINT('',(3.,-3.67394039744206E-16,6.1));
#138578=CARTESIAN_POINT('Origin',(0.,0.,6.1));
#138579=CARTESIAN_POINT('',(3.,-3.67394039744206E-16,6.7));
#138580=CARTESIAN_POINT('',(3.,-3.67394039744206E-16,0.));
#138581=CARTESIAN_POINT('Origin',(0.,0.,6.7));
#138582=CARTESIAN_POINT('',(2.93938769133981,0.6,6.1));
#138583=CARTESIAN_POINT('Origin',(0.,0.,6.1));
#138584=CARTESIAN_POINT('',(2.93938769133981,0.6,0.));
#138585=CARTESIAN_POINT('',(0.6,2.93938769133981,6.1));
#138586=CARTESIAN_POINT('',(0.6,2.93938769133981,0.));
#138587=CARTESIAN_POINT('',(-0.6,2.93938769133981,6.1));
#138588=CARTESIAN_POINT('Origin',(0.,0.,6.1));
#138589=CARTESIAN_POINT('',(-0.6,2.93938769133981,0.));
#138590=CARTESIAN_POINT('',(-2.93938769133981,0.6,6.1));
#138591=CARTESIAN_POINT('',(-2.93938769133981,0.6,0.));
#138592=CARTESIAN_POINT('',(-2.93938769133981,-0.6,6.1));
#138593=CARTESIAN_POINT('Origin',(0.,0.,6.1));
#138594=CARTESIAN_POINT('',(-2.93938769133981,-0.6,0.));
#138595=CARTESIAN_POINT('',(-0.6,-2.93938769133981,6.1));
#138596=CARTESIAN_POINT('',(-0.6,-2.93938769133981,0.));
#138597=CARTESIAN_POINT('',(0.6,-2.93938769133981,6.1));
#138598=CARTESIAN_POINT('Origin',(0.,0.,6.1));
#138599=CARTESIAN_POINT('',(0.6,-2.93938769133981,0.));
#138600=CARTESIAN_POINT('',(2.93938769133981,-0.6,0.));
#138601=CARTESIAN_POINT('Origin',(3.,0.,6.7));
#138602=CARTESIAN_POINT('',(5.,-6.12323399573677E-16,6.7));
#138603=CARTESIAN_POINT('Origin',(0.,0.,6.7));
#138604=CARTESIAN_POINT('Origin',(0.,0.,0.));
#138605=CARTESIAN_POINT('',(5.,-6.12323399573677E-16,8.));
#138606=CARTESIAN_POINT('',(5.,-6.12323399573677E-16,0.));
#138607=CARTESIAN_POINT('Origin',(0.,0.,8.));
#138608=CARTESIAN_POINT('Origin',(5.,0.,8.));
#138609=CARTESIAN_POINT('Origin',(1.90787840283389,0.6,6.1));
#138610=CARTESIAN_POINT('',(1.90787840283389,0.6,6.1));
#138611=CARTESIAN_POINT('Origin',(5.,-0.6,6.1));
#138612=CARTESIAN_POINT('',(5.,-0.6,6.1));
#138613=CARTESIAN_POINT('Origin',(0.,0.,6.1));
#138614=CARTESIAN_POINT('Origin',(-0.6,1.90787840283389,6.1));
#138615=CARTESIAN_POINT('',(-0.6,1.90787840283389,6.1));
#138616=CARTESIAN_POINT('Origin',(0.6,5.,6.1));
#138617=CARTESIAN_POINT('',(0.6,5.,6.1));
#138618=CARTESIAN_POINT('Origin',(0.,0.,6.1));
#138619=CARTESIAN_POINT('Origin',(-0.6,-5.,6.1));
#138620=CARTESIAN_POINT('',(-0.6,-5.,6.1));
#138621=CARTESIAN_POINT('Origin',(0.6,-1.90787840283389,6.1));
#138622=CARTESIAN_POINT('',(0.6,-1.90787840283389,6.1));
#138623=CARTESIAN_POINT('Origin',(0.,0.,6.1));
#138624=CARTESIAN_POINT('Origin',(-5.,0.6,6.1));
#138625=CARTESIAN_POINT('',(-5.,0.6,6.1));
#138626=CARTESIAN_POINT('Origin',(-1.90787840283389,-0.6,6.1));
#138627=CARTESIAN_POINT('',(-1.90787840283389,-0.6,6.1));
#138628=CARTESIAN_POINT('Origin',(0.,0.,6.1));
#138629=CARTESIAN_POINT('Origin',(2.7,1.89736659610103,6.7));
#138630=CARTESIAN_POINT('',(2.3,1.89736659610103,5.2));
#138631=CARTESIAN_POINT('',(2.37272727272727,1.6673827662706,5.2));
#138632=CARTESIAN_POINT('Origin',(2.7,1.89736659610103,5.2));
#138633=CARTESIAN_POINT('',(2.37272727272727,1.6673827662706,6.7));
#138634=CARTESIAN_POINT('',(2.37272727272727,1.6673827662706,6.7));
#138635=CARTESIAN_POINT('',(2.3,1.89736659610103,6.7));
#138636=CARTESIAN_POINT('Origin',(2.7,1.89736659610103,6.7));
#138637=CARTESIAN_POINT('',(2.3,1.89736659610103,6.7));
#138638=CARTESIAN_POINT('Origin',(2.3,1.76635217326557,6.7));
#138639=CARTESIAN_POINT('',(2.3,3.41064510027062,6.7));
#138640=CARTESIAN_POINT('',(2.3,1.76635217326557,6.7));
#138641=CARTESIAN_POINT('',(2.3,3.41064510027062,5.2));
#138642=CARTESIAN_POINT('',(2.3,3.41064510027062,6.7));
#138643=CARTESIAN_POINT('',(2.3,1.76635217326557,5.2));
#138644=CARTESIAN_POINT('Origin',(-3.26886955020535E-16,-1.42199013476836,
6.7));
#138645=CARTESIAN_POINT('',(-2.37272727272727,1.6673827662706,6.7));
#138646=CARTESIAN_POINT('Origin',(-1.534807777198E-23,0.,6.7));
#138647=CARTESIAN_POINT('',(-2.3,1.89736659610103,6.7));
#138648=CARTESIAN_POINT('Origin',(-2.7,1.89736659610103,6.7));
#138649=CARTESIAN_POINT('',(-2.3,3.41064510027062,6.7));
#138650=CARTESIAN_POINT('',(-2.3,1.76635217326557,6.7));
#138651=CARTESIAN_POINT('',(-2.94827586206897,3.72426763822654,6.7));
#138652=CARTESIAN_POINT('Origin',(-2.7,3.41064510027062,6.7));
#138653=CARTESIAN_POINT('',(-2.8,-3.83699100858993,6.7));
#138654=CARTESIAN_POINT('Origin',(-1.534807777198E-23,0.,6.7));
#138655=CARTESIAN_POINT('',(-2.8,-5.2,6.7));
#138656=CARTESIAN_POINT('',(-2.8,-7.,6.7));
#138657=CARTESIAN_POINT('',(2.8,-5.2,6.7));
#138658=CARTESIAN_POINT('',(1.4,-5.2,6.7));
#138659=CARTESIAN_POINT('',(2.8,-3.83699100858994,6.7));
#138660=CARTESIAN_POINT('',(2.8,-7.,6.7));
#138661=CARTESIAN_POINT('',(2.94827586206897,3.72426763822654,6.7));
#138662=CARTESIAN_POINT('Origin',(-1.534807777198E-23,0.,6.7));
#138663=CARTESIAN_POINT('Origin',(2.7,3.41064510027062,6.7));
#138664=CARTESIAN_POINT('Origin',(2.7,3.41064510027062,6.7));
#138665=CARTESIAN_POINT('',(2.94827586206897,3.72426763822654,5.2));
#138666=CARTESIAN_POINT('Origin',(2.7,3.41064510027062,5.2));
#138667=CARTESIAN_POINT('',(2.94827586206897,3.72426763822654,6.7));
#138668=CARTESIAN_POINT('Origin',(-1.534807777198E-23,0.,6.7));
#138669=CARTESIAN_POINT('',(2.8,-3.83699100858994,5.2));
#138670=CARTESIAN_POINT('',(2.8,-3.83699100858994,6.7));
#138671=CARTESIAN_POINT('Origin',(-1.534807777198E-23,0.,5.2));
#138672=CARTESIAN_POINT('Origin',(-2.7,1.89736659610103,6.7));
#138673=CARTESIAN_POINT('',(-2.37272727272727,1.6673827662706,5.2));
#138674=CARTESIAN_POINT('',(-2.3,1.89736659610103,5.2));
#138675=CARTESIAN_POINT('Origin',(-2.7,1.89736659610103,5.2));
#138676=CARTESIAN_POINT('',(-2.3,1.89736659610103,6.7));
#138677=CARTESIAN_POINT('',(-2.37272727272727,1.6673827662706,6.7));
#138678=CARTESIAN_POINT('Origin',(-1.534807777198E-23,0.,6.7));
#138679=CARTESIAN_POINT('Origin',(-1.534807777198E-23,0.,5.2));
#138680=CARTESIAN_POINT('Origin',(-2.7,3.41064510027062,6.7));
#138681=CARTESIAN_POINT('',(-2.3,3.41064510027062,5.2));
#138682=CARTESIAN_POINT('',(-2.94827586206897,3.72426763822654,5.2));
#138683=CARTESIAN_POINT('Origin',(-2.7,3.41064510027062,5.2));
#138684=CARTESIAN_POINT('',(-2.94827586206897,3.72426763822654,6.7));
#138685=CARTESIAN_POINT('',(-2.3,3.41064510027062,6.7));
#138686=CARTESIAN_POINT('Origin',(-1.534807777198E-23,0.,6.7));
#138687=CARTESIAN_POINT('',(-2.8,-3.83699100858993,5.2));
#138688=CARTESIAN_POINT('Origin',(-1.534807777198E-23,0.,5.2));
#138689=CARTESIAN_POINT('',(-2.8,-3.83699100858993,6.7));
#138690=CARTESIAN_POINT('Origin',(2.8,-5.2,6.7));
#138691=CARTESIAN_POINT('',(-2.8,-5.2,8.5));
#138692=CARTESIAN_POINT('',(-2.8,-5.2,6.7));
#138693=CARTESIAN_POINT('',(2.8,-5.2,8.5));
#138694=CARTESIAN_POINT('',(-2.8,-5.2,8.5));
#138695=CARTESIAN_POINT('',(2.8,-5.2,6.7));
#138696=CARTESIAN_POINT('Origin',(-1.84889274661175E-31,-6.1,8.5));
#138697=CARTESIAN_POINT('',(-2.8,-7.,8.5));
#138698=CARTESIAN_POINT('',(-2.8,-7.,8.5));
#138699=CARTESIAN_POINT('',(2.8,-7.,8.5));
#138700=CARTESIAN_POINT('',(-2.8,-7.,8.5));
#138701=CARTESIAN_POINT('',(2.8,-7.,8.5));
#138702=CARTESIAN_POINT('Origin',(2.8,-7.,6.7));
#138703=CARTESIAN_POINT('',(-2.8,-7.,5.2));
#138704=CARTESIAN_POINT('',(-2.8,-7.,6.7));
#138705=CARTESIAN_POINT('',(2.8,-7.,5.2));
#138706=CARTESIAN_POINT('',(-2.8,-7.,5.2));
#138707=CARTESIAN_POINT('',(2.8,-7.,6.7));
#138708=CARTESIAN_POINT('Origin',(2.8,-3.83699100858994,6.7));
#138709=CARTESIAN_POINT('',(2.8,-7.,5.2));
#138710=CARTESIAN_POINT('Origin',(-2.3,4.15601973046327,6.7));
#138711=CARTESIAN_POINT('',(-2.3,1.76635217326557,5.2));
#138712=CARTESIAN_POINT('Origin',(-2.8,-7.,6.7));
#138713=CARTESIAN_POINT('',(-2.8,-7.,5.2));
#138714=CARTESIAN_POINT('Origin',(-3.26886955020535E-16,-1.42199013476836,
5.2));
#459194=UNCERTAINTY_MEASURE_WITH_UNIT(LENGTH_MEASURE(0.01),#459243,
'DISTANCE_ACCURACY_VALUE',
'Maximum model space distance between geometric entities at asserted c
onnectivities');
#459216=UNCERTAINTY_MEASURE_WITH_UNIT(LENGTH_MEASURE(0.01),#459243,
'DISTANCE_ACCURACY_VALUE',
'Maximum model space distance between geometric entities at asserted c
onnectivities');
#459220=(
GEOMETRIC_REPRESENTATION_CONTEXT(3)
GLOBAL_UNCERTAINTY_ASSIGNED_CONTEXT((#459194))
GLOBAL_UNIT_ASSIGNED_CONTEXT((#459243,#459245,#459246))
REPRESENTATION_CONTEXT('','3D')
);
#459242=(
GEOMETRIC_REPRESENTATION_CONTEXT(3)
GLOBAL_UNCERTAINTY_ASSIGNED_CONTEXT((#459216))
GLOBAL_UNIT_ASSIGNED_CONTEXT((#459243,#459245,#459246))
REPRESENTATION_CONTEXT('','3D')
);
#459243=(
LENGTH_UNIT()
NAMED_UNIT(*)
SI_UNIT(.MILLI.,.METRE.)
);
#459245=(
NAMED_UNIT(*)
PLANE_ANGLE_UNIT()
SI_UNIT($,.RADIAN.)
);
#459246=(
NAMED_UNIT(*)
SI_UNIT($,.STERADIAN.)
SOLID_ANGLE_UNIT()
);
#459250=SHAPE_DEFINITION_REPRESENTATION(#459275,#459331);
#459275=PRODUCT_DEFINITION_SHAPE('',$,#459357);
#459331=SHAPE_REPRESENTATION('',(#95243),#459220);
#459353=PRODUCT_DEFINITION_CONTEXT('part definition',#459430,'design');
#459357=PRODUCT_DEFINITION('Pneumatic Adapter','Pneumatic Adapter',#459382,
#459353);
#459382=PRODUCT_DEFINITION_FORMATION('',$,#459435);
#459430=APPLICATION_CONTEXT(
'Core Data for Automotive Mechanical Design Process');
#459431=PRODUCT_CONTEXT('part definition',#459430,'mechanical');
#459435=PRODUCT('Pneumatic Adapter','Pneumatic Adapter',$,(#459431));
#459513=COLOUR_RGB('Sky Blue',0.24,0.69,0.87);
#459514=FILL_AREA_STYLE_COLOUR('',#459513);
#459515=FILL_AREA_STYLE('',(#459514));
#459516=SURFACE_STYLE_FILL_AREA(#459515);
#459517=SURFACE_SIDE_STYLE('',(#459516));
#459518=SURFACE_STYLE_USAGE(.BOTH.,#459517);
#459519=PRESENTATION_STYLE_ASSIGNMENT((#459518));
ENDSEC;
END-ISO-10303-21;
